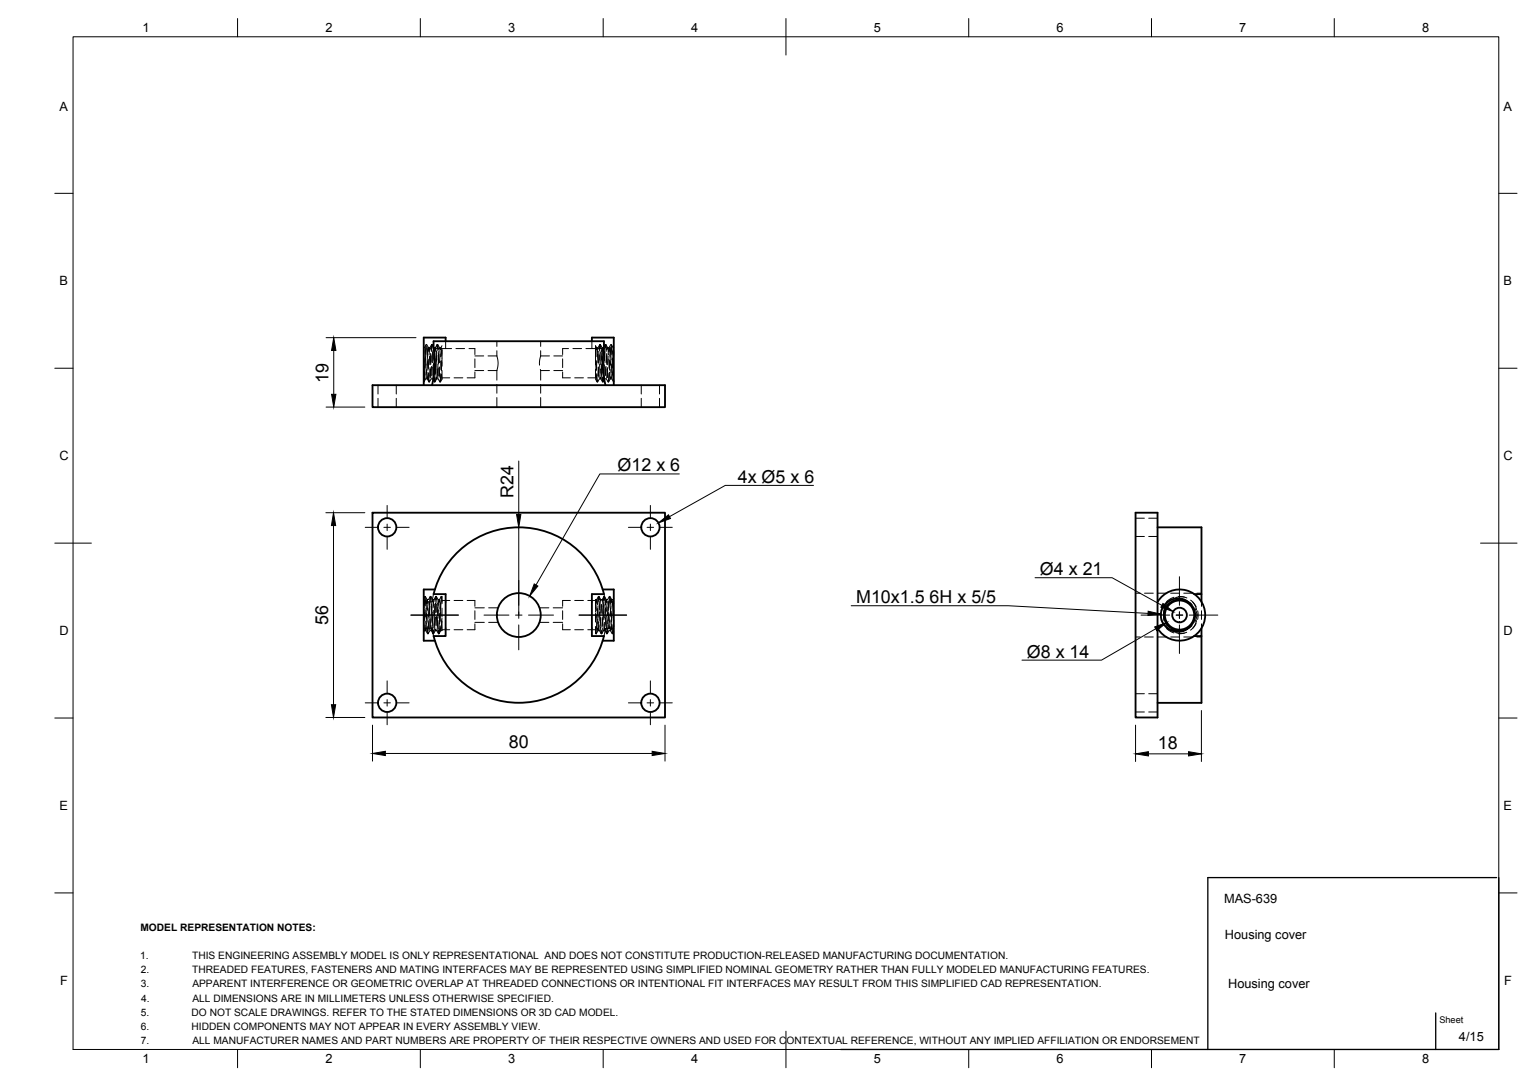
ISO-10303-21;
HEADER;
/* Generated by software containing ST-Developer
 * from STEP Tools, Inc. (www.steptools.com) 
 */

FILE_DESCRIPTION(
/* description */ ('Independent maintained push-to-latch/pull-to-reset mushroom-operator 
CAD. Two opposed spring-loaded ball detents in turned circular seats b
ias both travel stops; direct normally-closed bridge opens6mm when pre
ssed. Rounded palm/pull rim, captured head screw, removable detent clo
sures, native Coil spring families, insulated shared terminals and ord
inary machining features. Manual geometric states and ideal same-mater
ial spring-energy direction only; no electrical/safety certification, 
force/contact dynamics, wear, load or life rating. Requested blue/gray
 visual palette, not safety identification. External wiring/anchors an
d application engineering omitted.'),
/* implementation_level */ '2;1');

FILE_NAME(
/* name */ 'Housing cover.step',
/* time_stamp */ '2026-11-08T17:54:26-08:00',
/* author */ (''),
/* organization */ (''),
/* preprocessor_version */ 'ST-DEVELOPER v20.2',
/* originating_system */ 'Autodesk Translation Framework v15.17.0.0',
/* authorisation */ '');

FILE_SCHEMA (('AUTOMOTIVE_DESIGN { 1 0 10303 214 3 1 1 }'));
ENDSEC;

DATA;
#10=MECHANICAL_DESIGN_GEOMETRIC_PRESENTATION_REPRESENTATION('',(#191),#43980);
#157=SHAPE_REPRESENTATION_RELATIONSHIP('SRR','None',#44057,#174);
#174=ADVANCED_BREP_SHAPE_REPRESENTATION('',(#208),#43964);
#191=STYLED_ITEM('',(#44151),#208);
#208=MANIFOLD_SOLID_BREP('Body1',#11232);
#232=B_SPLINE_SURFACE_WITH_KNOTS('',3,3,((#23003,#23004,#23005,#23006,#23007,
#23008,#23009,#23010,#23011,#23012,#23013,#23014,#23015,#23016,#23017,#23018,
#23019,#23020,#23021,#23022,#23023,#23024,#23025,#23026,#23027,#23028,#23029,
#23030,#23031,#23032,#23033,#23034,#23035,#23036,#23037,#23038,#23039,#23040,
#23041,#23042,#23043,#23044,#23045,#23046,#23047,#23048,#23049,#23050,#23051),
(#23052,#23053,#23054,#23055,#23056,#23057,#23058,#23059,#23060,#23061,
#23062,#23063,#23064,#23065,#23066,#23067,#23068,#23069,#23070,#23071,#23072,
#23073,#23074,#23075,#23076,#23077,#23078,#23079,#23080,#23081,#23082,#23083,
#23084,#23085,#23086,#23087,#23088,#23089,#23090,#23091,#23092,#23093,#23094,
#23095,#23096,#23097,#23098,#23099,#23100),(#23101,#23102,#23103,#23104,
#23105,#23106,#23107,#23108,#23109,#23110,#23111,#23112,#23113,#23114,#23115,
#23116,#23117,#23118,#23119,#23120,#23121,#23122,#23123,#23124,#23125,#23126,
#23127,#23128,#23129,#23130,#23131,#23132,#23133,#23134,#23135,#23136,#23137,
#23138,#23139,#23140,#23141,#23142,#23143,#23144,#23145,#23146,#23147,#23148,
#23149),(#23150,#23151,#23152,#23153,#23154,#23155,#23156,#23157,#23158,
#23159,#23160,#23161,#23162,#23163,#23164,#23165,#23166,#23167,#23168,#23169,
#23170,#23171,#23172,#23173,#23174,#23175,#23176,#23177,#23178,#23179,#23180,
#23181,#23182,#23183,#23184,#23185,#23186,#23187,#23188,#23189,#23190,#23191,
#23192,#23193,#23194,#23195,#23196,#23197,#23198)),.UNSPECIFIED.,.F.,.F.,
 .F.,(4,4),(4,1,1,1,1,1,1,1,1,1,1,1,1,1,1,1,1,1,1,1,1,1,1,1,1,1,1,1,1,1,
1,1,1,1,1,1,1,1,1,1,1,1,1,1,1,1,4),(0.,0.0965329650085055),(11.852942864427,
12.3521979234545,12.851452982482,13.3507080415095,13.849963100537,14.3492181595645,
14.848473218592,15.3477282776195,15.846983336647,16.3462383956745,16.845493454702,
17.3447485137295,17.844003572757,18.3432586317845,18.842513690812,19.3417687498395,
19.841023808867,20.3402788678945,20.839533926922,21.3387889859495,21.838044044977,
22.3372991040045,22.836554163032,23.3358092220595,23.835064281087,24.3343193401145,
24.833574399142,25.3328294581695,25.832084517197,26.3313395762245,26.830594635252,
27.3298496942795,27.829104753307,28.3283598123345,28.827614871362,29.3268699303895,
29.826124989417,30.3253800484445,30.824635107472,31.3238901664995,31.823145225527,
32.3224002845545,32.821655343582,33.3209104026095,33.820165461637,34.3194205206645,
34.818675579692),.UNSPECIFIED.);
#233=B_SPLINE_SURFACE_WITH_KNOTS('',3,3,((#23385,#23386,#23387,#23388,#23389,
#23390,#23391,#23392,#23393,#23394,#23395,#23396,#23397,#23398,#23399,#23400,
#23401,#23402,#23403,#23404,#23405,#23406,#23407,#23408,#23409,#23410,#23411,
#23412,#23413,#23414,#23415,#23416,#23417,#23418,#23419,#23420,#23421,#23422,
#23423,#23424,#23425,#23426,#23427,#23428,#23429,#23430,#23431,#23432,#23433),
(#23434,#23435,#23436,#23437,#23438,#23439,#23440,#23441,#23442,#23443,
#23444,#23445,#23446,#23447,#23448,#23449,#23450,#23451,#23452,#23453,#23454,
#23455,#23456,#23457,#23458,#23459,#23460,#23461,#23462,#23463,#23464,#23465,
#23466,#23467,#23468,#23469,#23470,#23471,#23472,#23473,#23474,#23475,#23476,
#23477,#23478,#23479,#23480,#23481,#23482),(#23483,#23484,#23485,#23486,
#23487,#23488,#23489,#23490,#23491,#23492,#23493,#23494,#23495,#23496,#23497,
#23498,#23499,#23500,#23501,#23502,#23503,#23504,#23505,#23506,#23507,#23508,
#23509,#23510,#23511,#23512,#23513,#23514,#23515,#23516,#23517,#23518,#23519,
#23520,#23521,#23522,#23523,#23524,#23525,#23526,#23527,#23528,#23529,#23530,
#23531),(#23532,#23533,#23534,#23535,#23536,#23537,#23538,#23539,#23540,
#23541,#23542,#23543,#23544,#23545,#23546,#23547,#23548,#23549,#23550,#23551,
#23552,#23553,#23554,#23555,#23556,#23557,#23558,#23559,#23560,#23561,#23562,
#23563,#23564,#23565,#23566,#23567,#23568,#23569,#23570,#23571,#23572,#23573,
#23574,#23575,#23576,#23577,#23578,#23579,#23580)),.UNSPECIFIED.,.F.,.F.,
 .F.,(4,4),(4,1,1,1,1,1,1,1,1,1,1,1,1,1,1,1,1,1,1,1,1,1,1,1,1,1,1,1,1,1,
1,1,1,1,1,1,1,1,1,1,1,1,1,1,1,1,4),(0.,0.0965329650085055),(14.399609326548,
14.8988643855755,15.398119444603,15.8973745036305,16.396629562658,16.8958846216855,
17.395139680713,17.8943947397405,18.393649798768,18.8929048577955,19.392159916823,
19.8914149758505,20.390670034878,20.8899250939055,21.389180152933,21.8884352119605,
22.387690270988,22.8869453300155,23.386200389043,23.8854554480705,24.384710507098,
24.8839655661255,25.383220625153,25.8824756841805,26.381730743208,26.8809858022355,
27.380240861263,27.8794959202905,28.378750979318,28.8780060383455,29.377261097373,
29.8765161564005,30.375771215428,30.8750262744555,31.374281333483,31.8735363925105,
32.372791451538,32.8720465105655,33.371301569593,33.8705566286205,34.369811687648,
34.8690667466755,35.368321805703,35.8675768647305,36.366831923758,36.8660869827855,
37.365342041813),.UNSPECIFIED.);
#234=B_SPLINE_SURFACE_WITH_KNOTS('',3,3,((#23796,#23797,#23798,#23799,#23800,
#23801,#23802,#23803,#23804,#23805,#23806,#23807,#23808,#23809,#23810,#23811,
#23812,#23813,#23814,#23815,#23816,#23817,#23818,#23819,#23820,#23821,#23822,
#23823,#23824,#23825,#23826,#23827,#23828,#23829,#23830,#23831,#23832,#23833,
#23834,#23835,#23836,#23837,#23838,#23839,#23840,#23841,#23842,#23843,#23844),
(#23845,#23846,#23847,#23848,#23849,#23850,#23851,#23852,#23853,#23854,
#23855,#23856,#23857,#23858,#23859,#23860,#23861,#23862,#23863,#23864,#23865,
#23866,#23867,#23868,#23869,#23870,#23871,#23872,#23873,#23874,#23875,#23876,
#23877,#23878,#23879,#23880,#23881,#23882,#23883,#23884,#23885,#23886,#23887,
#23888,#23889,#23890,#23891,#23892,#23893),(#23894,#23895,#23896,#23897,
#23898,#23899,#23900,#23901,#23902,#23903,#23904,#23905,#23906,#23907,#23908,
#23909,#23910,#23911,#23912,#23913,#23914,#23915,#23916,#23917,#23918,#23919,
#23920,#23921,#23922,#23923,#23924,#23925,#23926,#23927,#23928,#23929,#23930,
#23931,#23932,#23933,#23934,#23935,#23936,#23937,#23938,#23939,#23940,#23941,
#23942),(#23943,#23944,#23945,#23946,#23947,#23948,#23949,#23950,#23951,
#23952,#23953,#23954,#23955,#23956,#23957,#23958,#23959,#23960,#23961,#23962,
#23963,#23964,#23965,#23966,#23967,#23968,#23969,#23970,#23971,#23972,#23973,
#23974,#23975,#23976,#23977,#23978,#23979,#23980,#23981,#23982,#23983,#23984,
#23985,#23986,#23987,#23988,#23989,#23990,#23991)),.UNSPECIFIED.,.F.,.F.,
 .F.,(4,4),(4,1,1,1,1,1,1,1,1,1,1,1,1,1,1,1,1,1,1,1,1,1,1,1,1,1,1,1,1,1,
1,1,1,1,1,1,1,1,1,1,1,1,1,1,1,1,4),(0.,0.0965329650085055),(11.852942864427,
12.3521979234545,12.851452982482,13.3507080415095,13.849963100537,14.3492181595645,
14.848473218592,15.3477282776195,15.846983336647,16.3462383956745,16.845493454702,
17.3447485137295,17.844003572757,18.3432586317845,18.842513690812,19.3417687498395,
19.841023808867,20.3402788678945,20.839533926922,21.3387889859495,21.838044044977,
22.3372991040045,22.836554163032,23.3358092220595,23.835064281087,24.3343193401145,
24.833574399142,25.3328294581695,25.832084517197,26.3313395762245,26.830594635252,
27.3298496942795,27.829104753307,28.3283598123345,28.827614871362,29.3268699303895,
29.826124989417,30.3253800484445,30.824635107472,31.3238901664995,31.823145225527,
32.3224002845545,32.821655343582,33.3209104026095,33.820165461637,34.3194205206645,
34.818675579692),.UNSPECIFIED.);
#235=B_SPLINE_SURFACE_WITH_KNOTS('',3,3,((#24178,#24179,#24180,#24181,#24182,
#24183,#24184,#24185,#24186,#24187,#24188,#24189,#24190,#24191,#24192,#24193,
#24194,#24195,#24196,#24197,#24198,#24199,#24200,#24201,#24202,#24203,#24204,
#24205,#24206,#24207,#24208,#24209,#24210,#24211,#24212,#24213,#24214,#24215,
#24216,#24217,#24218,#24219,#24220,#24221,#24222,#24223,#24224,#24225,#24226),
(#24227,#24228,#24229,#24230,#24231,#24232,#24233,#24234,#24235,#24236,
#24237,#24238,#24239,#24240,#24241,#24242,#24243,#24244,#24245,#24246,#24247,
#24248,#24249,#24250,#24251,#24252,#24253,#24254,#24255,#24256,#24257,#24258,
#24259,#24260,#24261,#24262,#24263,#24264,#24265,#24266,#24267,#24268,#24269,
#24270,#24271,#24272,#24273,#24274,#24275),(#24276,#24277,#24278,#24279,
#24280,#24281,#24282,#24283,#24284,#24285,#24286,#24287,#24288,#24289,#24290,
#24291,#24292,#24293,#24294,#24295,#24296,#24297,#24298,#24299,#24300,#24301,
#24302,#24303,#24304,#24305,#24306,#24307,#24308,#24309,#24310,#24311,#24312,
#24313,#24314,#24315,#24316,#24317,#24318,#24319,#24320,#24321,#24322,#24323,
#24324),(#24325,#24326,#24327,#24328,#24329,#24330,#24331,#24332,#24333,
#24334,#24335,#24336,#24337,#24338,#24339,#24340,#24341,#24342,#24343,#24344,
#24345,#24346,#24347,#24348,#24349,#24350,#24351,#24352,#24353,#24354,#24355,
#24356,#24357,#24358,#24359,#24360,#24361,#24362,#24363,#24364,#24365,#24366,
#24367,#24368,#24369,#24370,#24371,#24372,#24373)),.UNSPECIFIED.,.F.,.F.,
 .F.,(4,4),(4,1,1,1,1,1,1,1,1,1,1,1,1,1,1,1,1,1,1,1,1,1,1,1,1,1,1,1,1,1,
1,1,1,1,1,1,1,1,1,1,1,1,1,1,1,1,4),(0.,0.0965329650085055),(14.399609326548,
14.8988643855755,15.398119444603,15.8973745036305,16.396629562658,16.8958846216855,
17.395139680713,17.8943947397405,18.393649798768,18.8929048577955,19.392159916823,
19.8914149758505,20.390670034878,20.8899250939055,21.389180152933,21.8884352119605,
22.387690270988,22.8869453300155,23.386200389043,23.8854554480705,24.384710507098,
24.8839655661255,25.383220625153,25.8824756841805,26.381730743208,26.8809858022355,
27.380240861263,27.8794959202905,28.378750979318,28.8780060383455,29.377261097373,
29.8765161564005,30.375771215428,30.8750262744555,31.374281333483,31.8735363925105,
32.372791451538,32.8720465105655,33.371301569593,33.8705566286205,34.369811687648,
34.8690667466755,35.368321805703,35.8675768647305,36.366831923758,36.8660869827855,
37.365342041813),.UNSPECIFIED.);
#277=FACE_BOUND('',#1308,.T.);
#278=FACE_BOUND('',#1318,.T.);
#279=FACE_BOUND('',#1321,.T.);
#280=FACE_BOUND('',#1326,.T.);
#281=FACE_BOUND('',#1328,.T.);
#282=FACE_BOUND('',#1329,.T.);
#283=FACE_BOUND('',#1330,.T.);
#284=FACE_BOUND('',#1331,.T.);
#285=FACE_BOUND('',#1332,.T.);
#286=FACE_BOUND('',#1336,.T.);
#287=FACE_BOUND('',#1339,.T.);
#288=FACE_BOUND('',#1342,.T.);
#289=FACE_BOUND('',#1350,.T.);
#290=FACE_BOUND('',#1356,.T.);
#291=FACE_BOUND('',#1357,.T.);
#292=FACE_BOUND('',#1358,.T.);
#293=FACE_BOUND('',#1359,.T.);
#294=FACE_BOUND('',#1360,.T.);
#362=PLANE('',#11659);
#363=PLANE('',#11661);
#364=PLANE('',#11663);
#365=PLANE('',#11664);
#366=PLANE('',#11665);
#367=PLANE('',#11667);
#368=PLANE('',#11668);
#369=PLANE('',#11669);
#370=PLANE('',#11671);
#371=PLANE('',#11675);
#372=PLANE('',#11680);
#373=PLANE('',#11684);
#374=PLANE('',#11690);
#375=PLANE('',#11691);
#376=PLANE('',#11692);
#377=PLANE('',#11701);
#378=PLANE('',#11705);
#379=PLANE('',#11708);
#380=PLANE('',#11722);
#381=PLANE('',#11723);
#382=PLANE('',#11724);
#383=PLANE('',#11725);
#384=PLANE('',#11726);
#644=FACE_OUTER_BOUND('',#1285,.T.);
#645=FACE_OUTER_BOUND('',#1286,.T.);
#646=FACE_OUTER_BOUND('',#1287,.T.);
#647=FACE_OUTER_BOUND('',#1288,.T.);
#648=FACE_OUTER_BOUND('',#1289,.T.);
#649=FACE_OUTER_BOUND('',#1290,.T.);
#650=FACE_OUTER_BOUND('',#1291,.T.);
#651=FACE_OUTER_BOUND('',#1292,.T.);
#652=FACE_OUTER_BOUND('',#1293,.T.);
#653=FACE_OUTER_BOUND('',#1294,.T.);
#654=FACE_OUTER_BOUND('',#1295,.T.);
#655=FACE_OUTER_BOUND('',#1296,.T.);
#656=FACE_OUTER_BOUND('',#1297,.T.);
#657=FACE_OUTER_BOUND('',#1298,.T.);
#658=FACE_OUTER_BOUND('',#1299,.T.);
#659=FACE_OUTER_BOUND('',#1300,.T.);
#660=FACE_OUTER_BOUND('',#1301,.T.);
#661=FACE_OUTER_BOUND('',#1302,.T.);
#662=FACE_OUTER_BOUND('',#1303,.T.);
#663=FACE_OUTER_BOUND('',#1304,.T.);
#664=FACE_OUTER_BOUND('',#1305,.T.);
#665=FACE_OUTER_BOUND('',#1306,.T.);
#666=FACE_OUTER_BOUND('',#1307,.T.);
#667=FACE_OUTER_BOUND('',#1309,.T.);
#668=FACE_OUTER_BOUND('',#1310,.T.);
#669=FACE_OUTER_BOUND('',#1311,.T.);
#670=FACE_OUTER_BOUND('',#1312,.T.);
#671=FACE_OUTER_BOUND('',#1313,.T.);
#672=FACE_OUTER_BOUND('',#1314,.T.);
#673=FACE_OUTER_BOUND('',#1315,.T.);
#674=FACE_OUTER_BOUND('',#1316,.T.);
#675=FACE_OUTER_BOUND('',#1317,.T.);
#676=FACE_OUTER_BOUND('',#1319,.T.);
#677=FACE_OUTER_BOUND('',#1320,.T.);
#678=FACE_OUTER_BOUND('',#1322,.T.);
#679=FACE_OUTER_BOUND('',#1323,.T.);
#680=FACE_OUTER_BOUND('',#1324,.T.);
#681=FACE_OUTER_BOUND('',#1325,.T.);
#682=FACE_OUTER_BOUND('',#1327,.T.);
#683=FACE_OUTER_BOUND('',#1333,.T.);
#684=FACE_OUTER_BOUND('',#1334,.T.);
#685=FACE_OUTER_BOUND('',#1335,.T.);
#686=FACE_OUTER_BOUND('',#1337,.T.);
#687=FACE_OUTER_BOUND('',#1338,.T.);
#688=FACE_OUTER_BOUND('',#1340,.T.);
#689=FACE_OUTER_BOUND('',#1341,.T.);
#690=FACE_OUTER_BOUND('',#1343,.T.);
#691=FACE_OUTER_BOUND('',#1344,.T.);
#692=FACE_OUTER_BOUND('',#1345,.T.);
#693=FACE_OUTER_BOUND('',#1346,.T.);
#694=FACE_OUTER_BOUND('',#1347,.T.);
#695=FACE_OUTER_BOUND('',#1348,.T.);
#696=FACE_OUTER_BOUND('',#1349,.T.);
#697=FACE_OUTER_BOUND('',#1351,.T.);
#698=FACE_OUTER_BOUND('',#1352,.T.);
#699=FACE_OUTER_BOUND('',#1353,.T.);
#700=FACE_OUTER_BOUND('',#1354,.T.);
#701=FACE_OUTER_BOUND('',#1355,.T.);
#1285=EDGE_LOOP('',(#7755,#7756,#7757,#7758));
#1286=EDGE_LOOP('',(#7759,#7760,#7761,#7762));
#1287=EDGE_LOOP('',(#7763,#7764,#7765,#7766));
#1288=EDGE_LOOP('',(#7767,#7768,#7769,#7770));
#1289=EDGE_LOOP('',(#7771,#7772,#7773,#7774));
#1290=EDGE_LOOP('',(#7775,#7776,#7777,#7778));
#1291=EDGE_LOOP('',(#7779,#7780,#7781,#7782));
#1292=EDGE_LOOP('',(#7783,#7784,#7785,#7786));
#1293=EDGE_LOOP('',(#7787,#7788,#7789,#7790));
#1294=EDGE_LOOP('',(#7791,#7792,#7793,#7794));
#1295=EDGE_LOOP('',(#7795,#7796,#7797,#7798));
#1296=EDGE_LOOP('',(#7799,#7800,#7801,#7802));
#1297=EDGE_LOOP('',(#7803,#7804,#7805,#7806));
#1298=EDGE_LOOP('',(#7807,#7808,#7809,#7810));
#1299=EDGE_LOOP('',(#7811,#7812,#7813));
#1300=EDGE_LOOP('',(#7814,#7815,#7816));
#1301=EDGE_LOOP('',(#7817,#7818,#7819,#7820));
#1302=EDGE_LOOP('',(#7821,#7822,#7823,#7824));
#1303=EDGE_LOOP('',(#7825,#7826,#7827));
#1304=EDGE_LOOP('',(#7828,#7829,#7830,#7831));
#1305=EDGE_LOOP('',(#7832,#7833,#7834,#7835));
#1306=EDGE_LOOP('',(#7836,#7837,#7838));
#1307=EDGE_LOOP('',(#7839,#7840,#7841,#7842,#7843,#7844,#7845,#7846,#7847,
#7848,#7849,#7850));
#1308=EDGE_LOOP('',(#7851));
#1309=EDGE_LOOP('',(#7852,#7853));
#1310=EDGE_LOOP('',(#7854,#7855,#7856,#7857));
#1311=EDGE_LOOP('',(#7858,#7859,#7860,#7861,#7862,#7863,#7864,#7865,#7866,
#7867,#7868));
#1312=EDGE_LOOP('',(#7869,#7870,#7871,#7872,#7873,#7874,#7875,#7876,#7877,
#7878,#7879));
#1313=EDGE_LOOP('',(#7880,#7881,#7882,#7883));
#1314=EDGE_LOOP('',(#7884,#7885,#7886,#7887,#7888,#7889,#7890,#7891,#7892,
#7893,#7894));
#1315=EDGE_LOOP('',(#7895,#7896,#7897,#7898,#7899,#7900,#7901,#7902,#7903,
#7904,#7905));
#1316=EDGE_LOOP('',(#7906,#7907,#7908,#7909));
#1317=EDGE_LOOP('',(#7910,#7911,#7912,#7913));
#1318=EDGE_LOOP('',(#7914));
#1319=EDGE_LOOP('',(#7915,#7916,#7917,#7918));
#1320=EDGE_LOOP('',(#7919));
#1321=EDGE_LOOP('',(#7920));
#1322=EDGE_LOOP('',(#7921,#7922,#7923,#7924,#7925));
#1323=EDGE_LOOP('',(#7926,#7927,#7928,#7929,#7930,#7931,#7932,#7933,#7934,
#7935));
#1324=EDGE_LOOP('',(#7936,#7937));
#1325=EDGE_LOOP('',(#7938,#7939));
#1326=EDGE_LOOP('',(#7940,#7941,#7942,#7943));
#1327=EDGE_LOOP('',(#7944,#7945,#7946,#7947));
#1328=EDGE_LOOP('',(#7948));
#1329=EDGE_LOOP('',(#7949));
#1330=EDGE_LOOP('',(#7950));
#1331=EDGE_LOOP('',(#7951));
#1332=EDGE_LOOP('',(#7952,#7953,#7954,#7955,#7956,#7957,#7958,#7959));
#1333=EDGE_LOOP('',(#7960,#7961,#7962,#7963,#7964,#7965));
#1334=EDGE_LOOP('',(#7966,#7967,#7968,#7969));
#1335=EDGE_LOOP('',(#7970,#7971,#7972,#7973));
#1336=EDGE_LOOP('',(#7974));
#1337=EDGE_LOOP('',(#7975,#7976,#7977,#7978));
#1338=EDGE_LOOP('',(#7979));
#1339=EDGE_LOOP('',(#7980));
#1340=EDGE_LOOP('',(#7981,#7982,#7983,#7984,#7985,#7986,#7987));
#1341=EDGE_LOOP('',(#7988,#7989));
#1342=EDGE_LOOP('',(#7990,#7991,#7992,#7993));
#1343=EDGE_LOOP('',(#7994,#7995,#7996,#7997,#7998,#7999,#8000,#8001,#8002,
#8003));
#1344=EDGE_LOOP('',(#8004,#8005,#8006,#8007,#8008,#8009));
#1345=EDGE_LOOP('',(#8010,#8011,#8012,#8013));
#1346=EDGE_LOOP('',(#8014,#8015,#8016,#8017));
#1347=EDGE_LOOP('',(#8018,#8019,#8020,#8021));
#1348=EDGE_LOOP('',(#8022,#8023,#8024,#8025));
#1349=EDGE_LOOP('',(#8026,#8027,#8028,#8029,#8030,#8031,#8032,#8033,#8034,
#8035));
#1350=EDGE_LOOP('',(#8036,#8037));
#1351=EDGE_LOOP('',(#8038,#8039,#8040,#8041));
#1352=EDGE_LOOP('',(#8042,#8043,#8044,#8045));
#1353=EDGE_LOOP('',(#8046,#8047,#8048,#8049));
#1354=EDGE_LOOP('',(#8050,#8051,#8052,#8053));
#1355=EDGE_LOOP('',(#8054,#8055,#8056,#8057));
#1356=EDGE_LOOP('',(#8058));
#1357=EDGE_LOOP('',(#8059));
#1358=EDGE_LOOP('',(#8060));
#1359=EDGE_LOOP('',(#8061));
#1360=EDGE_LOOP('',(#8062));
#1847=CIRCLE('',#11638,0.4263);
#1848=CIRCLE('',#11641,0.4263);
#1849=CIRCLE('',#11643,0.4263);
#1850=CIRCLE('',#11646,0.4263);
#1851=CIRCLE('',#11648,0.5099);
#1852=CIRCLE('',#11652,0.5099);
#1853=CIRCLE('',#11654,0.5099);
#1854=CIRCLE('',#11658,0.5099);
#1855=CIRCLE('',#11660,0.7);
#1856=CIRCLE('',#11662,0.7);
#1857=CIRCLE('',#11666,0.7);
#1858=CIRCLE('',#11670,0.7);
#1859=CIRCLE('',#11672,2.4);
#1860=CIRCLE('',#11673,2.4);
#1861=CIRCLE('',#11674,0.6);
#1862=CIRCLE('',#11676,0.7);
#1863=CIRCLE('',#11681,0.4);
#1864=CIRCLE('',#11683,0.4);
#1865=CIRCLE('',#11685,0.2);
#1866=CIRCLE('',#11688,0.7);
#1867=CIRCLE('',#11689,0.7);
#1868=CIRCLE('',#11693,0.25);
#1869=CIRCLE('',#11694,0.25);
#1870=CIRCLE('',#11695,0.25);
#1871=CIRCLE('',#11696,0.25);
#1872=CIRCLE('',#11697,2.4);
#1873=CIRCLE('',#11698,2.4);
#1874=CIRCLE('',#11702,0.4);
#1875=CIRCLE('',#11704,0.4);
#1876=CIRCLE('',#11706,0.2);
#1877=CIRCLE('',#11709,0.7);
#1878=CIRCLE('',#11713,0.25);
#1879=CIRCLE('',#11715,0.25);
#1880=CIRCLE('',#11717,0.25);
#1881=CIRCLE('',#11719,0.25);
#1882=CIRCLE('',#11721,0.6);
#2228=B_SPLINE_CURVE_WITH_KNOTS('',3,(#22266,#22267,#22268,#22269,#22270,
#22271,#22272,#22273,#22274,#22275,#22276,#22277,#22278,#22279,#22280,#22281,
#22282,#22283,#22284),.UNSPECIFIED.,.F.,.F.,(4,3,3,3,3,3,4),(20.1579098629397,
20.4694574201275,20.968712479155,21.4679675381825,21.96722259721,22.4664776562375,
22.965732715265),.UNSPECIFIED.);
#2229=B_SPLINE_CURVE_WITH_KNOTS('',3,(#22287,#22288,#22289,#22290,#22291,
#22292,#22293,#22294,#22295,#22296,#22297,#22298,#22299,#22300,#22301,#22302,
#22303,#22304,#22305,#22306,#22307,#22308,#22309,#22310,#22311,#22312,#22313,
#22314,#22315,#22316,#22317),.UNSPECIFIED.,.F.,.F.,(4,3,3,3,3,3,3,3,3,3,
4),(-20.9439510239319,-20.4694574201275,-19.9702023611,-19.4709473020725,
-18.971692243045,-18.4724371840175,-17.97318212499,-17.4739270659625,-16.974672006935,
-16.4754169479075,-16.4213910178811),.UNSPECIFIED.);
#2230=B_SPLINE_CURVE_WITH_KNOTS('',3,(#22322,#22323,#22324,#22325,#22326,
#22327,#22328,#22329,#22330,#22331,#22332,#22333,#22334,#22335,#22336,#22337,
#22338,#22339,#22340,#22341,#22342,#22343,#22344,#22345,#22346,#22347,#22348,
#22349,#22350,#22351,#22352,#22353,#22354,#22355,#22356,#22357,#22358,#22359,
#22360,#22361,#22362,#22363,#22364),.UNSPECIFIED.,.F.,.F.,(4,3,3,3,3,3,
3,3,3,3,3,3,3,3,4),(13.8747245557602,13.97914165277,14.4783967117975,14.977651770825,
15.4769068298525,15.97616188888,16.4754169479075,16.974672006935,17.4739270659625,
17.97318212499,18.4724371840175,18.971692243045,19.4709473020725,19.9702023611,
20.1579098629397),.UNSPECIFIED.);
#2231=B_SPLINE_CURVE_WITH_KNOTS('',3,(#22365,#22366,#22367,#22368,#22369,
#22370,#22371,#22372,#22373,#22374,#22375,#22376,#22377,#22378,#22379,#22380,
#22381,#22382,#22383,#22384,#22385,#22386,#22387,#22388,#22389,#22390,#22391,
#22392,#22393,#22394,#22395,#22396,#22397,#22398,#22399,#22400,#22401,#22402,
#22403,#22404),.UNSPECIFIED.,.F.,.F.,(4,3,3,3,3,3,3,3,3,3,3,3,3,4),(-16.4213910178811,
-15.97616188888,-15.4769068298525,-14.977651770825,-14.4783967117975,-13.97914165277,
-13.4798865937425,-12.980631534715,-12.4813764756875,-11.98212141666,-11.4828663576325,
-10.983611298605,-10.4843562395775,-10.1382057107016),.UNSPECIFIED.);
#2232=B_SPLINE_CURVE_WITH_KNOTS('',3,(#22410,#22411,#22412,#22413,#22414,
#22415,#22416,#22417,#22418,#22419,#22420,#22421,#22422,#22423,#22424,#22425,
#22426,#22427,#22428,#22429,#22430,#22431,#22432,#22433,#22434),
 .UNSPECIFIED.,.F.,.F.,(4,3,3,3,3,3,3,3,4),(-3.85502040352197,-3.49478541319251,
-2.995530354165,-2.4962752951375,-1.99702023611001,-1.4977651770825,-0.998510118055002,
-0.499255059027501,0.),.UNSPECIFIED.);
#2233=B_SPLINE_CURVE_WITH_KNOTS('',3,(#22437,#22438,#22439,#22440,#22441,
#22442,#22443,#22444,#22445,#22446,#22447,#22448,#22449,#22450,#22451,#22452,
#22453,#22454,#22455,#22456,#22457,#22458,#22459,#22460,#22461,#22462,#22463,
#22464,#22465,#22466,#22467,#22468,#22469,#22470,#22471,#22472,#22473),
 .UNSPECIFIED.,.F.,.F.,(4,3,3,3,3,3,3,3,3,3,3,3,4),(2.02178169133306,2.4962752951375,
2.99553035416501,3.49478541319251,3.99404047222001,4.49329553124751,4.99255059027501,
5.49180564930251,5.99106070833001,6.49031576735751,6.98957082638501,7.48882588541252,
7.59153924858057),.UNSPECIFIED.);
#2234=B_SPLINE_CURVE_WITH_KNOTS('',3,(#22479,#22480,#22481,#22482,#22483,
#22484,#22485,#22486,#22487,#22488,#22489,#22490,#22491,#22492,#22493,#22494,
#22495,#22496,#22497),.UNSPECIFIED.,.F.,.F.,(4,3,3,3,3,3,4),(20.1579098629397,
20.4694574201275,20.968712479155,21.4679675381825,21.96722259721,22.4664776562375,
22.965732715265),.UNSPECIFIED.);
#2235=B_SPLINE_CURVE_WITH_KNOTS('',3,(#22500,#22501,#22502,#22503,#22504,
#22505,#22506,#22507,#22508,#22509,#22510,#22511,#22512,#22513,#22514,#22515,
#22516,#22517,#22518,#22519,#22520,#22521,#22522,#22523,#22524,#22525,#22526,
#22527,#22528,#22529,#22530),.UNSPECIFIED.,.F.,.F.,(4,3,3,3,3,3,3,3,3,3,
4),(-20.9439510239319,-20.4694574201275,-19.9702023611,-19.4709473020725,
-18.971692243045,-18.4724371840175,-17.97318212499,-17.4739270659625,-16.974672006935,
-16.4754169479075,-16.4213910178811),.UNSPECIFIED.);
#2236=B_SPLINE_CURVE_WITH_KNOTS('',3,(#22535,#22536,#22537,#22538,#22539,
#22540,#22541,#22542,#22543,#22544,#22545,#22546,#22547,#22548,#22549,#22550,
#22551,#22552,#22553,#22554,#22555,#22556,#22557,#22558,#22559,#22560,#22561,
#22562,#22563,#22564,#22565,#22566,#22567,#22568,#22569,#22570,#22571,#22572,
#22573,#22574,#22575,#22576,#22577),.UNSPECIFIED.,.F.,.F.,(4,3,3,3,3,3,
3,3,3,3,3,3,3,3,4),(13.8747245557602,13.97914165277,14.4783967117975,14.977651770825,
15.4769068298525,15.97616188888,16.4754169479075,16.974672006935,17.4739270659625,
17.97318212499,18.4724371840175,18.971692243045,19.4709473020725,19.9702023611,
20.1579098629397),.UNSPECIFIED.);
#2237=B_SPLINE_CURVE_WITH_KNOTS('',3,(#22578,#22579,#22580,#22581,#22582,
#22583,#22584,#22585,#22586,#22587,#22588,#22589,#22590,#22591,#22592,#22593,
#22594,#22595,#22596,#22597,#22598,#22599,#22600,#22601,#22602,#22603,#22604,
#22605,#22606,#22607,#22608,#22609,#22610,#22611,#22612,#22613,#22614,#22615,
#22616,#22617),.UNSPECIFIED.,.F.,.F.,(4,3,3,3,3,3,3,3,3,3,3,3,3,4),(-16.4213910178811,
-15.97616188888,-15.4769068298525,-14.977651770825,-14.4783967117975,-13.97914165277,
-13.4798865937425,-12.980631534715,-12.4813764756875,-11.98212141666,-11.4828663576325,
-10.983611298605,-10.4843562395775,-10.1382057107016),.UNSPECIFIED.);
#2238=B_SPLINE_CURVE_WITH_KNOTS('',3,(#22623,#22624,#22625,#22626,#22627,
#22628,#22629,#22630,#22631,#22632,#22633,#22634,#22635,#22636,#22637,#22638,
#22639,#22640,#22641,#22642,#22643,#22644,#22645,#22646,#22647),
 .UNSPECIFIED.,.F.,.F.,(4,3,3,3,3,3,3,3,4),(-3.85502040352197,-3.49478541319251,
-2.995530354165,-2.4962752951375,-1.99702023611001,-1.4977651770825,-0.998510118055002,
-0.499255059027501,0.),.UNSPECIFIED.);
#2239=B_SPLINE_CURVE_WITH_KNOTS('',3,(#22650,#22651,#22652,#22653,#22654,
#22655,#22656,#22657,#22658,#22659,#22660,#22661,#22662,#22663,#22664,#22665,
#22666,#22667,#22668,#22669,#22670,#22671,#22672,#22673,#22674,#22675,#22676,
#22677,#22678,#22679,#22680,#22681,#22682,#22683,#22684,#22685,#22686),
 .UNSPECIFIED.,.F.,.F.,(4,3,3,3,3,3,3,3,3,3,3,3,4),(2.02178169133306,2.4962752951375,
2.99553035416501,3.49478541319251,3.99404047222001,4.49329553124751,4.99255059027501,
5.49180564930251,5.99106070833001,6.49031576735751,6.98957082638501,7.48882588541252,
7.59153924858057),.UNSPECIFIED.);
#2240=B_SPLINE_CURVE_WITH_KNOTS('',3,(#22692,#22693,#22694,#22695),
 .UNSPECIFIED.,.F.,.F.,(4,4),(34.5575191894877,34.818675579692),
 .UNSPECIFIED.);
#2241=B_SPLINE_CURVE_WITH_KNOTS('',3,(#22698,#22699,#22700,#22701,#22702),
 .UNSPECIFIED.,.F.,.F.,(4,1,4),(34.5575191894877,34.8690667466755,35.3435603504799),
 .UNSPECIFIED.);
#2242=B_SPLINE_CURVE_WITH_KNOTS('',3,(#22707,#22708,#22709,#22710,#22711,
#22712,#22713,#22714,#22715,#22716,#22717,#22718,#22719,#22720,#22721,#22722,
#22723),.UNSPECIFIED.,.F.,.F.,(4,1,1,1,1,1,1,1,1,1,1,1,1,1,4),(28.2743338823081,
28.3283598123345,28.827614871362,29.3268699303895,29.826124989417,30.3253800484445,
30.824635107472,31.3238901664995,31.823145225527,32.3224002845545,32.821655343582,
33.3209104026095,33.820165461637,34.3194205206645,34.5575191894877),
 .UNSPECIFIED.);
#2243=B_SPLINE_CURVE_WITH_KNOTS('',3,(#22724,#22725,#22726,#22727,#22728,
#22729,#22730,#22731,#22732,#22733,#22734,#22735,#22736,#22737,#22738,#22739,
#22740),.UNSPECIFIED.,.F.,.F.,(4,1,1,1,1,1,1,1,1,1,1,1,1,1,4),(28.2743338823081,
28.378750979318,28.8780060383455,29.377261097373,29.8765161564005,30.375771215428,
30.8750262744555,31.374281333483,31.8735363925105,32.372791451538,32.8720465105655,
33.371301569593,33.8705566286205,34.369811687648,34.5575191894877),
 .UNSPECIFIED.);
#2244=B_SPLINE_CURVE_WITH_KNOTS('',3,(#22745,#22746,#22747,#22748,#22749,
#22750,#22751,#22752,#22753,#22754,#22755,#22756,#22757,#22758,#22759,#22760),
 .UNSPECIFIED.,.F.,.F.,(4,1,1,1,1,1,1,1,1,1,1,1,1,4),(21.9911485751285,
22.3372991040045,22.836554163032,23.3358092220595,23.835064281087,24.3343193401145,
24.833574399142,25.3328294581695,25.832084517197,26.3313395762245,26.830594635252,
27.3298496942795,27.829104753307,28.2743338823081),.UNSPECIFIED.);
#2245=B_SPLINE_CURVE_WITH_KNOTS('',3,(#22761,#22762,#22763,#22764,#22765,
#22766,#22767,#22768,#22769,#22770,#22771,#22772,#22773,#22774,#22775,#22776),
 .UNSPECIFIED.,.F.,.F.,(4,1,1,1,1,1,1,1,1,1,1,1,1,4),(21.9911485751285,
22.387690270988,22.8869453300155,23.386200389043,23.8854554480705,24.384710507098,
24.8839655661255,25.383220625153,25.8824756841805,26.381730743208,26.8809858022355,
27.380240861263,27.8794959202905,28.2743338823081),.UNSPECIFIED.);
#2246=B_SPLINE_CURVE_WITH_KNOTS('',3,(#22782,#22783,#22784,#22785,#22786,
#22787),.UNSPECIFIED.,.F.,.F.,(4,1,1,4),(14.399609326548,14.8988643855755,
15.398119444603,15.707963267949),.UNSPECIFIED.);
#2247=B_SPLINE_CURVE_WITH_KNOTS('',3,(#22790,#22791,#22792,#22793,#22794,
#22795,#22796),.UNSPECIFIED.,.F.,.F.,(4,1,1,1,4),(13.8747245557601,14.3492181595645,
14.848473218592,15.3477282776195,15.707963267949),.UNSPECIFIED.);
#2248=B_SPLINE_CURVE_WITH_KNOTS('',3,(#22802,#22803,#22804,#22805),
 .UNSPECIFIED.,.F.,.F.,(4,4),(34.5575191894877,34.818675579692),
 .UNSPECIFIED.);
#2249=B_SPLINE_CURVE_WITH_KNOTS('',3,(#22808,#22809,#22810,#22811,#22812),
 .UNSPECIFIED.,.F.,.F.,(4,1,4),(34.5575191894877,34.8690667466755,35.3435603504799),
 .UNSPECIFIED.);
#2250=B_SPLINE_CURVE_WITH_KNOTS('',3,(#22817,#22818,#22819,#22820,#22821,
#22822,#22823,#22824,#22825,#22826,#22827,#22828,#22829,#22830,#22831,#22832,
#22833),.UNSPECIFIED.,.F.,.F.,(4,1,1,1,1,1,1,1,1,1,1,1,1,1,4),(28.2743338823081,
28.3283598123345,28.827614871362,29.3268699303895,29.826124989417,30.3253800484445,
30.824635107472,31.3238901664995,31.823145225527,32.3224002845545,32.821655343582,
33.3209104026095,33.820165461637,34.3194205206645,34.5575191894877),
 .UNSPECIFIED.);
#2251=B_SPLINE_CURVE_WITH_KNOTS('',3,(#22834,#22835,#22836,#22837,#22838,
#22839,#22840,#22841,#22842,#22843,#22844,#22845,#22846,#22847,#22848,#22849,
#22850),.UNSPECIFIED.,.F.,.F.,(4,1,1,1,1,1,1,1,1,1,1,1,1,1,4),(28.2743338823081,
28.378750979318,28.8780060383455,29.377261097373,29.8765161564005,30.375771215428,
30.8750262744555,31.374281333483,31.8735363925105,32.372791451538,32.8720465105655,
33.371301569593,33.8705566286205,34.369811687648,34.5575191894877),
 .UNSPECIFIED.);
#2252=B_SPLINE_CURVE_WITH_KNOTS('',3,(#22855,#22856,#22857,#22858,#22859,
#22860,#22861,#22862,#22863,#22864,#22865,#22866,#22867,#22868,#22869,#22870),
 .UNSPECIFIED.,.F.,.F.,(4,1,1,1,1,1,1,1,1,1,1,1,1,4),(21.9911485751285,
22.3372991040045,22.836554163032,23.3358092220595,23.835064281087,24.3343193401145,
24.833574399142,25.3328294581695,25.832084517197,26.3313395762245,26.830594635252,
27.3298496942795,27.829104753307,28.2743338823081),.UNSPECIFIED.);
#2253=B_SPLINE_CURVE_WITH_KNOTS('',3,(#22871,#22872,#22873,#22874,#22875,
#22876,#22877,#22878,#22879,#22880,#22881,#22882,#22883,#22884,#22885,#22886),
 .UNSPECIFIED.,.F.,.F.,(4,1,1,1,1,1,1,1,1,1,1,1,1,4),(21.9911485751285,
22.387690270988,22.8869453300155,23.386200389043,23.8854554480705,24.384710507098,
24.8839655661255,25.383220625153,25.8824756841805,26.381730743208,26.8809858022355,
27.380240861263,27.8794959202905,28.2743338823081),.UNSPECIFIED.);
#2254=B_SPLINE_CURVE_WITH_KNOTS('',3,(#22892,#22893,#22894,#22895,#22896,
#22897),.UNSPECIFIED.,.F.,.F.,(4,1,1,4),(14.399609326548,14.8988643855755,
15.398119444603,15.707963267949),.UNSPECIFIED.);
#2255=B_SPLINE_CURVE_WITH_KNOTS('',3,(#22900,#22901,#22902,#22903,#22904,
#22905,#22906),.UNSPECIFIED.,.F.,.F.,(4,1,1,1,4),(13.8747245557601,14.3492181595645,
14.848473218592,15.3477282776195,15.707963267949),.UNSPECIFIED.);
#2256=B_SPLINE_CURVE_WITH_KNOTS('',3,(#22969,#22970,#22971,#22972,#22973,
#22974,#22975,#22976,#22977,#22978,#22979,#22980,#22981,#22982,#22983,#22984,
#22985),.UNSPECIFIED.,.F.,.F.,(4,1,1,1,1,1,1,1,1,1,1,1,1,1,4),(15.707963267949,
15.846983336647,16.3462383956745,16.845493454702,17.3447485137295,17.844003572757,
18.3432586317845,18.842513690812,19.3417687498395,19.841023808867,20.3402788678945,
20.839533926922,21.3387889859495,21.838044044977,21.9911485751285),
 .UNSPECIFIED.);
#2257=B_SPLINE_CURVE_WITH_KNOTS('',3,(#22986,#22987,#22988,#22989,#22990,
#22991,#22992,#22993,#22994,#22995,#22996,#22997,#22998,#22999,#23000,#23001,
#23002),.UNSPECIFIED.,.F.,.F.,(4,1,1,1,1,1,1,1,1,1,1,1,1,1,4),(15.707963267949,
15.8973745036305,16.396629562658,16.8958846216855,17.395139680713,17.8943947397405,
18.393649798768,18.8929048577955,19.392159916823,19.8914149758505,20.390670034878,
20.8899250939055,21.389180152933,21.8884352119605,21.9911485751285),
 .UNSPECIFIED.);
#2258=B_SPLINE_CURVE_WITH_KNOTS('',3,(#23199,#23200,#23201,#23202,#23203,
#23204,#23205,#23206,#23207,#23208,#23209,#23210,#23211,#23212,#23213,#23214,
#23215,#23216,#23217,#23218,#23219,#23220,#23221,#23222,#23223,#23224,#23225,
#23226,#23227,#23228,#23229,#23230,#23231,#23232,#23233,#23234,#23235,#23236,
#23237,#23238,#23239,#23240,#23241,#23242,#23243,#23244,#23245,#23246,#23247,
#23248,#23249,#23250,#23251,#23252,#23253,#23254,#23255,#23256,#23257,#23258,
#23259,#23260,#23261,#23262,#23263,#23264,#23265,#23266,#23267,#23268,#23269,
#23270,#23271),.UNSPECIFIED.,.F.,.F.,(4,3,3,3,3,3,3,3,3,3,3,3,3,3,3,3,3,
3,3,3,3,3,3,3,4),(-0.950777871811465,-0.888334407370769,-0.851051814776991,
-0.82737904373313,-0.764191528890905,-0.727096293545134,-0.707864357405063,
-0.701004014048681,-0.624532510230306,-0.548715306176616,-0.528886751702636,
-0.51335217329456,-0.460845815077925,-0.386468184274459,-0.349072714542667,
-0.331943455188318,-0.259671363135132,-0.230659644409349,-0.19743434794885,
-0.175120034180883,-0.157580682039417,-0.0841021758717334,-0.0150413926252008,
-0.0106236697040495,0.),.UNSPECIFIED.);
#2259=B_SPLINE_CURVE_WITH_KNOTS('',3,(#23272,#23273,#23274,#23275,#23276,
#23277,#23278,#23279,#23280,#23281,#23282,#23283,#23284,#23285,#23286,#23287,
#23288,#23289,#23290,#23291,#23292,#23293,#23294,#23295,#23296,#23297,#23298,
#23299,#23300,#23301,#23302,#23303,#23304,#23305,#23306,#23307,#23308,#23309,
#23310,#23311,#23312,#23313,#23314,#23315,#23316,#23317,#23318,#23319,#23320,
#23321,#23322,#23323,#23324,#23325,#23326,#23327,#23328,#23329,#23330,#23331,
#23332,#23333,#23334,#23335,#23336,#23337,#23338,#23339,#23340,#23341),
 .UNSPECIFIED.,.F.,.F.,(4,3,3,3,3,3,3,3,3,3,3,3,3,3,3,3,3,3,3,3,3,3,3,4),
(0.,0.0695167991119783,0.140212658431775,0.162172470483188,0.179979408684031,
0.219498223261391,0.291822018016311,0.337745303611425,0.355228583776568,
0.429645631566202,0.449180111380345,0.509263572656178,0.525649154341391,
0.601088264154331,0.677503858556246,0.688874999321038,0.709603483853625,
0.730479306054779,0.782399641108501,0.820902701806524,0.845385896033558,
0.924612288143001,0.938160646269666,0.950777871811463),.UNSPECIFIED.);
#2260=B_SPLINE_CURVE_WITH_KNOTS('',3,(#23342,#23343,#23344,#23345,#23346,
#23347,#23348,#23349,#23350,#23351,#23352,#23353,#23354,#23355,#23356,#23357,
#23358,#23359,#23360,#23361,#23362,#23363,#23364,#23365,#23366,#23367,#23368,
#23369,#23370,#23371,#23372,#23373,#23374,#23375,#23376,#23377,#23378,#23379,
#23380,#23381,#23382,#23383,#23384),.UNSPECIFIED.,.F.,.F.,(4,3,3,3,3,3,
3,3,3,3,3,3,3,3,4),(-10.1382057107016,-9.98510118055001,-9.48584612152251,
-8.98659106249501,-8.48733600346751,-7.98808094444001,-7.48882588541251,
-6.98957082638501,-6.49031576735751,-5.99106070833001,-5.49180564930251,
-4.99255059027501,-4.49329553124751,-3.99404047222001,-3.85502040352197),
 .UNSPECIFIED.);
#2261=B_SPLINE_CURVE_WITH_KNOTS('',3,(#23581,#23582,#23583,#23584,#23585,
#23586,#23587,#23588,#23589,#23590,#23591,#23592,#23593,#23594,#23595,#23596,
#23597,#23598,#23599,#23600,#23601,#23602,#23603,#23604,#23605,#23606,#23607,
#23608,#23609,#23610,#23611,#23612,#23613,#23614,#23615,#23616,#23617,#23618,
#23619,#23620,#23621,#23622,#23623,#23624,#23625,#23626,#23627,#23628,#23629,
#23630,#23631,#23632,#23633,#23634,#23635,#23636,#23637,#23638,#23639,#23640,
#23641,#23642,#23643,#23644,#23645,#23646,#23647,#23648,#23649,#23650),
 .UNSPECIFIED.,.F.,.F.,(4,3,3,3,3,3,3,3,3,3,3,3,3,3,3,3,3,3,3,3,3,3,3,4),
(-0.954382097139049,-0.899410408801335,-0.859358635307587,-0.836685957905282,
-0.785590650846737,-0.75140161257743,-0.734495343788191,-0.662158982507963,
-0.588787990221564,-0.570217280263643,-0.551422718402641,-0.504011712732237,
-0.443843717567291,-0.393584703400901,-0.372143080358795,-0.295059059270718,
-0.263339732072452,-0.224912725821683,-0.201648013648112,-0.183362315801792,
-0.105092336646239,-0.0261711118220366,-0.0126626251736613,0.),
 .UNSPECIFIED.);
#2262=B_SPLINE_CURVE_WITH_KNOTS('',3,(#23651,#23652,#23653,#23654,#23655,
#23656,#23657,#23658,#23659,#23660,#23661,#23662,#23663,#23664,#23665,#23666,
#23667,#23668,#23669,#23670,#23671,#23672,#23673,#23674,#23675,#23676,#23677,
#23678,#23679,#23680,#23681,#23682,#23683,#23684,#23685,#23686,#23687,#23688,
#23689,#23690),.UNSPECIFIED.,.F.,.F.,(4,3,3,3,3,3,3,3,3,3,3,3,3,4),(7.59153924858057,
7.98808094444002,8.48733600346752,8.98659106249502,9.48584612152252,9.98510118055002,
10.4843562395775,10.983611298605,11.4828663576325,11.98212141666,12.4813764756875,
12.980631534715,13.4798865937425,13.8747245557602),.UNSPECIFIED.);
#2263=B_SPLINE_CURVE_WITH_KNOTS('',3,(#23691,#23692,#23693,#23694,#23695,
#23696,#23697,#23698,#23699,#23700,#23701,#23702,#23703,#23704,#23705,#23706,
#23707,#23708,#23709,#23710,#23711,#23712,#23713,#23714,#23715,#23716,#23717,
#23718,#23719,#23720,#23721,#23722,#23723,#23724,#23725,#23726,#23727,#23728,
#23729,#23730,#23731,#23732,#23733,#23734,#23735,#23736,#23737,#23738,#23739,
#23740,#23741,#23742,#23743,#23744,#23745,#23746,#23747,#23748,#23749,#23750,
#23751,#23752,#23753,#23754,#23755,#23756,#23757,#23758,#23759,#23760),
 .UNSPECIFIED.,.F.,.F.,(4,3,3,3,3,3,3,3,3,3,3,3,3,3,3,3,3,3,3,3,3,3,3,4),
(0.,0.079016546580938,0.157641122394585,0.183993443720854,0.207891281656444,
0.251131687956984,0.328243571587973,0.374168384090539,0.397099877179475,
0.472026294619315,0.492301725366521,0.550056206928688,0.568103933485432,
0.584735378149958,0.65759847554391,0.72331965161519,0.743939980328521,0.763679188248337,
0.809798919188833,0.846311488438111,0.867561854219163,0.937273050771799,
0.943726018375008,0.954382097139032),.UNSPECIFIED.);
#2264=B_SPLINE_CURVE_WITH_KNOTS('',3,(#23762,#23763,#23764,#23765,#23766,
#23767,#23768,#23769,#23770,#23771,#23772,#23773,#23774,#23775,#23776,#23777,
#23778),.UNSPECIFIED.,.F.,.F.,(4,1,1,1,1,1,1,1,1,1,1,1,1,1,4),(15.707963267949,
15.846983336647,16.3462383956745,16.845493454702,17.3447485137295,17.844003572757,
18.3432586317845,18.842513690812,19.3417687498395,19.841023808867,20.3402788678945,
20.839533926922,21.3387889859495,21.838044044977,21.9911485751285),
 .UNSPECIFIED.);
#2265=B_SPLINE_CURVE_WITH_KNOTS('',3,(#23779,#23780,#23781,#23782,#23783,
#23784,#23785,#23786,#23787,#23788,#23789,#23790,#23791,#23792,#23793,#23794,
#23795),.UNSPECIFIED.,.F.,.F.,(4,1,1,1,1,1,1,1,1,1,1,1,1,1,4),(15.707963267949,
15.8973745036305,16.396629562658,16.8958846216855,17.395139680713,17.8943947397405,
18.393649798768,18.8929048577955,19.392159916823,19.8914149758505,20.390670034878,
20.8899250939055,21.389180152933,21.8884352119605,21.9911485751285),
 .UNSPECIFIED.);
#2266=B_SPLINE_CURVE_WITH_KNOTS('',3,(#23992,#23993,#23994,#23995,#23996,
#23997,#23998,#23999,#24000,#24001,#24002,#24003,#24004,#24005,#24006,#24007,
#24008,#24009,#24010,#24011,#24012,#24013,#24014,#24015,#24016,#24017,#24018,
#24019,#24020,#24021,#24022,#24023,#24024,#24025,#24026,#24027,#24028,#24029,
#24030,#24031,#24032,#24033,#24034,#24035,#24036,#24037,#24038,#24039,#24040,
#24041,#24042,#24043,#24044,#24045,#24046,#24047,#24048,#24049,#24050,#24051,
#24052,#24053,#24054,#24055,#24056,#24057,#24058,#24059,#24060,#24061,#24062,
#24063,#24064),.UNSPECIFIED.,.F.,.F.,(4,3,3,3,3,3,3,3,3,3,3,3,3,3,3,3,3,
3,3,3,3,3,3,3,4),(-0.950777871811465,-0.888334407370769,-0.851051814776991,
-0.82737904373313,-0.764191528890905,-0.727096293545134,-0.707864357405063,
-0.701004014048681,-0.624532510230306,-0.548715306176616,-0.528886751702636,
-0.51335217329456,-0.460845815077925,-0.386468184274459,-0.349072714542667,
-0.331943455188318,-0.259671363135132,-0.230659644409349,-0.19743434794885,
-0.175120034180883,-0.157580682039417,-0.0841021758717334,-0.0150413926252008,
-0.0106236697040495,0.),.UNSPECIFIED.);
#2267=B_SPLINE_CURVE_WITH_KNOTS('',3,(#24065,#24066,#24067,#24068,#24069,
#24070,#24071,#24072,#24073,#24074,#24075,#24076,#24077,#24078,#24079,#24080,
#24081,#24082,#24083,#24084,#24085,#24086,#24087,#24088,#24089,#24090,#24091,
#24092,#24093,#24094,#24095,#24096,#24097,#24098,#24099,#24100,#24101,#24102,
#24103,#24104,#24105,#24106,#24107,#24108,#24109,#24110,#24111,#24112,#24113,
#24114,#24115,#24116,#24117,#24118,#24119,#24120,#24121,#24122,#24123,#24124,
#24125,#24126,#24127,#24128,#24129,#24130,#24131,#24132,#24133,#24134),
 .UNSPECIFIED.,.F.,.F.,(4,3,3,3,3,3,3,3,3,3,3,3,3,3,3,3,3,3,3,3,3,3,3,4),
(0.,0.0695167991119783,0.140212658431775,0.162172470483188,0.179979408684031,
0.219498223261391,0.291822018016311,0.337745303611425,0.355228583776568,
0.429645631566202,0.449180111380345,0.509263572656178,0.525649154341391,
0.601088264154331,0.677503858556246,0.688874999321038,0.709603483853625,
0.730479306054779,0.782399641108501,0.820902701806524,0.845385896033558,
0.924612288143001,0.938160646269666,0.950777871811463),.UNSPECIFIED.);
#2268=B_SPLINE_CURVE_WITH_KNOTS('',3,(#24135,#24136,#24137,#24138,#24139,
#24140,#24141,#24142,#24143,#24144,#24145,#24146,#24147,#24148,#24149,#24150,
#24151,#24152,#24153,#24154,#24155,#24156,#24157,#24158,#24159,#24160,#24161,
#24162,#24163,#24164,#24165,#24166,#24167,#24168,#24169,#24170,#24171,#24172,
#24173,#24174,#24175,#24176,#24177),.UNSPECIFIED.,.F.,.F.,(4,3,3,3,3,3,
3,3,3,3,3,3,3,3,4),(-10.1382057107016,-9.98510118055001,-9.48584612152251,
-8.98659106249501,-8.48733600346751,-7.98808094444001,-7.48882588541251,
-6.98957082638501,-6.49031576735751,-5.99106070833001,-5.49180564930251,
-4.99255059027501,-4.49329553124751,-3.99404047222001,-3.85502040352197),
 .UNSPECIFIED.);
#2269=B_SPLINE_CURVE_WITH_KNOTS('',3,(#24374,#24375,#24376,#24377,#24378,
#24379,#24380,#24381,#24382,#24383,#24384,#24385,#24386,#24387,#24388,#24389,
#24390,#24391,#24392,#24393,#24394,#24395,#24396,#24397,#24398,#24399,#24400,
#24401,#24402,#24403,#24404,#24405,#24406,#24407,#24408,#24409,#24410,#24411,
#24412,#24413,#24414,#24415,#24416,#24417,#24418,#24419,#24420,#24421,#24422,
#24423,#24424,#24425,#24426,#24427,#24428,#24429,#24430,#24431,#24432,#24433,
#24434,#24435,#24436,#24437,#24438,#24439,#24440,#24441,#24442,#24443),
 .UNSPECIFIED.,.F.,.F.,(4,3,3,3,3,3,3,3,3,3,3,3,3,3,3,3,3,3,3,3,3,3,3,4),
(-0.954382097139049,-0.899410408801335,-0.859358635307587,-0.836685957905282,
-0.785590650846737,-0.75140161257743,-0.734495343788191,-0.662158982507963,
-0.588787990221564,-0.570217280263643,-0.551422718402641,-0.504011712732237,
-0.443843717567291,-0.393584703400901,-0.372143080358795,-0.295059059270718,
-0.263339732072452,-0.224912725821683,-0.201648013648112,-0.183362315801792,
-0.105092336646239,-0.0261711118220366,-0.0126626251736613,0.),
 .UNSPECIFIED.);
#2270=B_SPLINE_CURVE_WITH_KNOTS('',3,(#24444,#24445,#24446,#24447,#24448,
#24449,#24450,#24451,#24452,#24453,#24454,#24455,#24456,#24457,#24458,#24459,
#24460,#24461,#24462,#24463,#24464,#24465,#24466,#24467,#24468,#24469,#24470,
#24471,#24472,#24473,#24474,#24475,#24476,#24477,#24478,#24479,#24480,#24481,
#24482,#24483),.UNSPECIFIED.,.F.,.F.,(4,3,3,3,3,3,3,3,3,3,3,3,3,4),(7.59153924858057,
7.98808094444002,8.48733600346752,8.98659106249502,9.48584612152252,9.98510118055002,
10.4843562395775,10.983611298605,11.4828663576325,11.98212141666,12.4813764756875,
12.980631534715,13.4798865937425,13.8747245557602),.UNSPECIFIED.);
#2271=B_SPLINE_CURVE_WITH_KNOTS('',3,(#24484,#24485,#24486,#24487,#24488,
#24489,#24490,#24491,#24492,#24493,#24494,#24495,#24496,#24497,#24498,#24499,
#24500,#24501,#24502,#24503,#24504,#24505,#24506,#24507,#24508,#24509,#24510,
#24511,#24512,#24513,#24514,#24515,#24516,#24517,#24518,#24519,#24520,#24521,
#24522,#24523,#24524,#24525,#24526,#24527,#24528,#24529,#24530,#24531,#24532,
#24533,#24534,#24535,#24536,#24537,#24538,#24539,#24540,#24541,#24542,#24543,
#24544,#24545,#24546,#24547,#24548,#24549,#24550,#24551,#24552,#24553),
 .UNSPECIFIED.,.F.,.F.,(4,3,3,3,3,3,3,3,3,3,3,3,3,3,3,3,3,3,3,3,3,3,3,4),
(0.,0.079016546580938,0.157641122394585,0.183993443720854,0.207891281656444,
0.251131687956984,0.328243571587973,0.374168384090539,0.397099877179475,
0.472026294619315,0.492301725366521,0.550056206928688,0.568103933485432,
0.584735378149958,0.65759847554391,0.72331965161519,0.743939980328521,0.763679188248337,
0.809798919188833,0.846311488438111,0.867561854219163,0.937273050771799,
0.943726018375008,0.954382097139032),.UNSPECIFIED.);
#2272=B_SPLINE_CURVE_WITH_KNOTS('',3,(#24569,#24570,#24571,#24572,#24573,
#24574,#24575,#24576,#24577,#24578,#24579,#24580,#24581,#24582,#24583,#24584,
#24585,#24586),.UNSPECIFIED.,.F.,.F.,(4,2,2,2,2,2,2,2,4),(0.,0.0759876362447371,
0.151975272489474,0.227927665609885,0.303880058730296,0.379832451850707,
0.455784844971118,0.531772481215855,0.607760117460592),.UNSPECIFIED.);
#2273=B_SPLINE_CURVE_WITH_KNOTS('',3,(#24587,#24588,#24589,#24590,#24591,
#24592,#24593,#24594,#24595,#24596,#24597,#24598,#24599,#24600,#24601,#24602,
#24603,#24604),.UNSPECIFIED.,.F.,.F.,(4,2,2,2,2,2,2,2,4),(0.607760117460592,
0.68374775370533,0.759735389950067,0.835687783070478,0.911640176190889,
0.9875925693113,1.06354496243171,1.13953259867645,1.21552023492118),
 .UNSPECIFIED.);
#2274=B_SPLINE_CURVE_WITH_KNOTS('',3,(#24609,#24610,#24611,#24612,#24613,
#24614,#24615,#24616,#24617,#24618,#24619,#24620,#24621),.UNSPECIFIED.,
 .F.,.F.,(4,2,3,2,2,4),(-0.408608378270607,-0.265388212066323,0.,0.265388212066323,
0.530776424132647,0.698056008856335),.UNSPECIFIED.);
#2275=B_SPLINE_CURVE_WITH_KNOTS('',3,(#24624,#24625,#24626,#24627,#24628,
#24629,#24630,#24631,#24632,#24633,#24634,#24635),.UNSPECIFIED.,.F.,.F.,
(4,2,2,2,2,4),(1.42476853019388,1.59204811491757,1.85743632698389,2.12282453905022,
2.38821275111654,2.53143291732083),.UNSPECIFIED.);
#2276=B_SPLINE_CURVE_WITH_KNOTS('',3,(#24669,#24670,#24671,#24672,#24673,
#24674,#24675,#24676,#24677,#24678,#24679,#24680,#24681),.UNSPECIFIED.,
 .F.,.F.,(4,2,3,2,2,4),(-0.408608378270607,-0.265388212066323,0.,0.265388212066323,
0.530776424132647,0.698056008856335),.UNSPECIFIED.);
#2277=B_SPLINE_CURVE_WITH_KNOTS('',3,(#24697,#24698,#24699,#24700,#24701,
#24702,#24703,#24704,#24705,#24706),.UNSPECIFIED.,.F.,.F.,(4,2,2,2,4),(0.303880058730296,
0.379832451850707,0.455784844971118,0.531772481215855,0.607760117460592),
 .UNSPECIFIED.);
#2278=B_SPLINE_CURVE_WITH_KNOTS('',3,(#24708,#24709,#24710,#24711,#24712,
#24713,#24714,#24715,#24716,#24717),.UNSPECIFIED.,.F.,.F.,(4,2,2,2,4),(0.,
0.0759876362447371,0.151975272489474,0.227927665609885,0.303880058730296),
 .UNSPECIFIED.);
#2279=B_SPLINE_CURVE_WITH_KNOTS('',3,(#24719,#24720,#24721,#24722,#24723,
#24724,#24725,#24726,#24727,#24728),.UNSPECIFIED.,.F.,.F.,(4,2,2,2,4),(0.911640176190889,
0.9875925693113,1.06354496243171,1.13953259867645,1.21552023492118),
 .UNSPECIFIED.);
#2280=B_SPLINE_CURVE_WITH_KNOTS('',3,(#24729,#24730,#24731,#24732,#24733,
#24734,#24735,#24736,#24737,#24738),.UNSPECIFIED.,.F.,.F.,(4,2,2,2,4),(0.607760117460592,
0.68374775370533,0.759735389950067,0.835687783070478,0.911640176190889),
 .UNSPECIFIED.);
#2281=B_SPLINE_CURVE_WITH_KNOTS('',3,(#24742,#24743,#24744,#24745,#24746,
#24747,#24748,#24749,#24750,#24751,#24752,#24753),.UNSPECIFIED.,.F.,.F.,
(4,2,2,2,2,4),(1.42476853019388,1.59204811491757,1.85743632698389,2.12282453905022,
2.38821275111654,2.53143291732083),.UNSPECIFIED.);
#2995=LINE('',#22264,#3627);
#2996=LINE('',#22321,#3628);
#2997=LINE('',#22408,#3629);
#2998=LINE('',#22477,#3630);
#2999=LINE('',#22534,#3631);
#3000=LINE('',#22621,#3632);
#3001=LINE('',#22690,#3633);
#3002=LINE('',#22706,#3634);
#3003=LINE('',#22744,#3635);
#3004=LINE('',#22780,#3636);
#3005=LINE('',#22800,#3637);
#3006=LINE('',#22816,#3638);
#3007=LINE('',#22854,#3639);
#3008=LINE('',#22890,#3640);
#3009=LINE('',#22912,#3641);
#3010=LINE('',#22913,#3642);
#3011=LINE('',#22919,#3643);
#3012=LINE('',#22920,#3644);
#3013=LINE('',#22924,#3645);
#3014=LINE('',#22926,#3646);
#3015=LINE('',#22928,#3647);
#3016=LINE('',#22929,#3648);
#3017=LINE('',#22933,#3649);
#3018=LINE('',#22935,#3650);
#3019=LINE('',#22937,#3651);
#3020=LINE('',#22938,#3652);
#3021=LINE('',#22942,#3653);
#3022=LINE('',#22945,#3654);
#3023=LINE('',#22947,#3655);
#3024=LINE('',#22948,#3656);
#3025=LINE('',#22951,#3657);
#3026=LINE('',#22953,#3658);
#3027=LINE('',#22954,#3659);
#3028=LINE('',#22958,#3660);
#3029=LINE('',#22960,#3661);
#3030=LINE('',#22962,#3662);
#3031=LINE('',#24560,#3663);
#3032=LINE('',#24567,#3664);
#3033=LINE('',#24608,#3665);
#3034=LINE('',#24637,#3666);
#3035=LINE('',#24641,#3667);
#3036=LINE('',#24645,#3668);
#3037=LINE('',#24647,#3669);
#3038=LINE('',#24649,#3670);
#3039=LINE('',#24650,#3671);
#3040=LINE('',#24662,#3672);
#3041=LINE('',#24664,#3673);
#3042=LINE('',#24666,#3674);
#3043=LINE('',#24688,#3675);
#3044=LINE('',#24695,#3676);
#3045=LINE('',#24757,#3677);
#3046=LINE('',#24761,#3678);
#3047=LINE('',#24765,#3679);
#3048=LINE('',#24769,#3680);
#3049=LINE('',#24772,#3681);
#3050=LINE('',#24774,#3682);
#3051=LINE('',#24779,#3683);
#3052=LINE('',#24780,#3684);
#3053=LINE('',#24781,#3685);
#3054=LINE('',#24784,#3686);
#3055=LINE('',#24785,#3687);
#3056=LINE('',#24788,#3688);
#3057=LINE('',#24789,#3689);
#3058=LINE('',#24791,#3690);
#3627=VECTOR('',#12836,0.5);
#3628=VECTOR('',#12841,0.5);
#3629=VECTOR('',#12844,0.5);
#3630=VECTOR('',#12849,0.5);
#3631=VECTOR('',#12854,0.5);
#3632=VECTOR('',#12857,0.5);
#3633=VECTOR('',#12862,0.5099);
#3634=VECTOR('',#12867,0.5099);
#3635=VECTOR('',#12870,0.5099);
#3636=VECTOR('',#12873,0.5099);
#3637=VECTOR('',#12878,0.5099);
#3638=VECTOR('',#12883,0.5099);
#3639=VECTOR('',#12886,0.5099);
#3640=VECTOR('',#12889,0.5099);
#3641=VECTOR('',#12896,1.);
#3642=VECTOR('',#12897,1.);
#3643=VECTOR('',#12902,1.);
#3644=VECTOR('',#12903,1.);
#3645=VECTOR('',#12906,1.);
#3646=VECTOR('',#12907,1.);
#3647=VECTOR('',#12908,1.);
#3648=VECTOR('',#12909,1.);
#3649=VECTOR('',#12912,1.);
#3650=VECTOR('',#12913,1.);
#3651=VECTOR('',#12914,1.);
#3652=VECTOR('',#12915,1.);
#3653=VECTOR('',#12920,1.);
#3654=VECTOR('',#12923,1.);
#3655=VECTOR('',#12924,1.);
#3656=VECTOR('',#12925,1.);
#3657=VECTOR('',#12928,1.);
#3658=VECTOR('',#12929,1.);
#3659=VECTOR('',#12930,1.);
#3660=VECTOR('',#12935,1.);
#3661=VECTOR('',#12938,1.);
#3662=VECTOR('',#12941,1.);
#3663=VECTOR('',#12962,0.4);
#3664=VECTOR('',#12971,0.2);
#3665=VECTOR('',#12974,1.);
#3666=VECTOR('',#12977,1.);
#3667=VECTOR('',#12984,1.);
#3668=VECTOR('',#12987,1.);
#3669=VECTOR('',#12988,1.);
#3670=VECTOR('',#12989,1.);
#3671=VECTOR('',#12990,1.);
#3672=VECTOR('',#13001,1.);
#3673=VECTOR('',#13002,1.);
#3674=VECTOR('',#13003,1.);
#3675=VECTOR('',#13016,0.4);
#3676=VECTOR('',#13025,0.2);
#3677=VECTOR('',#13036,0.25);
#3678=VECTOR('',#13041,0.25);
#3679=VECTOR('',#13046,0.25);
#3680=VECTOR('',#13051,0.25);
#3681=VECTOR('',#13056,0.6);
#3682=VECTOR('',#13057,0.6);
#3683=VECTOR('',#13062,1.);
#3684=VECTOR('',#13063,1.);
#3685=VECTOR('',#13064,1.);
#3686=VECTOR('',#13067,1.);
#3687=VECTOR('',#13068,1.);
#3688=VECTOR('',#13071,1.);
#3689=VECTOR('',#13072,1.);
#3690=VECTOR('',#13075,1.);
#4392=VERTEX_POINT('',#22262);
#4393=VERTEX_POINT('',#22263);
#4394=VERTEX_POINT('',#22265);
#4395=VERTEX_POINT('',#22285);
#4396=VERTEX_POINT('',#22319);
#4397=VERTEX_POINT('',#22320);
#4398=VERTEX_POINT('',#22406);
#4399=VERTEX_POINT('',#22407);
#4400=VERTEX_POINT('',#22409);
#4401=VERTEX_POINT('',#22435);
#4402=VERTEX_POINT('',#22475);
#4403=VERTEX_POINT('',#22476);
#4404=VERTEX_POINT('',#22478);
#4405=VERTEX_POINT('',#22498);
#4406=VERTEX_POINT('',#22532);
#4407=VERTEX_POINT('',#22533);
#4408=VERTEX_POINT('',#22619);
#4409=VERTEX_POINT('',#22620);
#4410=VERTEX_POINT('',#22622);
#4411=VERTEX_POINT('',#22648);
#4412=VERTEX_POINT('',#22688);
#4413=VERTEX_POINT('',#22689);
#4414=VERTEX_POINT('',#22691);
#4415=VERTEX_POINT('',#22696);
#4416=VERTEX_POINT('',#22704);
#4417=VERTEX_POINT('',#22705);
#4418=VERTEX_POINT('',#22742);
#4419=VERTEX_POINT('',#22743);
#4420=VERTEX_POINT('',#22778);
#4421=VERTEX_POINT('',#22779);
#4422=VERTEX_POINT('',#22781);
#4423=VERTEX_POINT('',#22788);
#4424=VERTEX_POINT('',#22798);
#4425=VERTEX_POINT('',#22799);
#4426=VERTEX_POINT('',#22801);
#4427=VERTEX_POINT('',#22806);
#4428=VERTEX_POINT('',#22814);
#4429=VERTEX_POINT('',#22815);
#4430=VERTEX_POINT('',#22852);
#4431=VERTEX_POINT('',#22853);
#4432=VERTEX_POINT('',#22888);
#4433=VERTEX_POINT('',#22889);
#4434=VERTEX_POINT('',#22891);
#4435=VERTEX_POINT('',#22898);
#4436=VERTEX_POINT('',#22908);
#4437=VERTEX_POINT('',#22909);
#4438=VERTEX_POINT('',#22911);
#4439=VERTEX_POINT('',#22915);
#4440=VERTEX_POINT('',#22916);
#4441=VERTEX_POINT('',#22918);
#4442=VERTEX_POINT('',#22922);
#4443=VERTEX_POINT('',#22923);
#4444=VERTEX_POINT('',#22925);
#4445=VERTEX_POINT('',#22927);
#4446=VERTEX_POINT('',#22931);
#4447=VERTEX_POINT('',#22932);
#4448=VERTEX_POINT('',#22934);
#4449=VERTEX_POINT('',#22936);
#4450=VERTEX_POINT('',#22940);
#4451=VERTEX_POINT('',#22944);
#4452=VERTEX_POINT('',#22946);
#4453=VERTEX_POINT('',#22950);
#4454=VERTEX_POINT('',#22952);
#4455=VERTEX_POINT('',#22956);
#4456=VERTEX_POINT('',#22964);
#4457=VERTEX_POINT('',#24556);
#4458=VERTEX_POINT('',#24559);
#4459=VERTEX_POINT('',#24563);
#4460=VERTEX_POINT('',#24566);
#4461=VERTEX_POINT('',#24568);
#4462=VERTEX_POINT('',#24606);
#4463=VERTEX_POINT('',#24607);
#4464=VERTEX_POINT('',#24623);
#4465=VERTEX_POINT('',#24636);
#4466=VERTEX_POINT('',#24643);
#4467=VERTEX_POINT('',#24644);
#4468=VERTEX_POINT('',#24646);
#4469=VERTEX_POINT('',#24648);
#4470=VERTEX_POINT('',#24651);
#4471=VERTEX_POINT('',#24653);
#4472=VERTEX_POINT('',#24655);
#4473=VERTEX_POINT('',#24657);
#4474=VERTEX_POINT('',#24659);
#4475=VERTEX_POINT('',#24661);
#4476=VERTEX_POINT('',#24663);
#4477=VERTEX_POINT('',#24665);
#4478=VERTEX_POINT('',#24684);
#4479=VERTEX_POINT('',#24687);
#4480=VERTEX_POINT('',#24691);
#4481=VERTEX_POINT('',#24694);
#4482=VERTEX_POINT('',#24696);
#4483=VERTEX_POINT('',#24707);
#4484=VERTEX_POINT('',#24718);
#4485=VERTEX_POINT('',#24756);
#4486=VERTEX_POINT('',#24760);
#4487=VERTEX_POINT('',#24764);
#4488=VERTEX_POINT('',#24768);
#4489=VERTEX_POINT('',#24773);
#4490=VERTEX_POINT('',#24777);
#4491=VERTEX_POINT('',#24778);
#4492=VERTEX_POINT('',#24783);
#4493=VERTEX_POINT('',#24787);
#5647=EDGE_CURVE('',#4392,#4393,#2995,.T.);
#5648=EDGE_CURVE('',#4393,#4394,#2228,.T.);
#5649=EDGE_CURVE('',#4394,#4395,#1847,.F.);
#5650=EDGE_CURVE('',#4395,#4392,#2229,.T.);
#5651=EDGE_CURVE('',#4396,#4397,#2996,.T.);
#5652=EDGE_CURVE('',#4397,#4393,#2230,.T.);
#5653=EDGE_CURVE('',#4392,#4396,#2231,.T.);
#5654=EDGE_CURVE('',#4398,#4399,#2997,.T.);
#5655=EDGE_CURVE('',#4398,#4400,#2232,.T.);
#5656=EDGE_CURVE('',#4401,#4400,#1848,.F.);
#5657=EDGE_CURVE('',#4401,#4399,#2233,.T.);
#5658=EDGE_CURVE('',#4402,#4403,#2998,.T.);
#5659=EDGE_CURVE('',#4403,#4404,#2234,.T.);
#5660=EDGE_CURVE('',#4404,#4405,#1849,.F.);
#5661=EDGE_CURVE('',#4405,#4402,#2235,.T.);
#5662=EDGE_CURVE('',#4406,#4407,#2999,.T.);
#5663=EDGE_CURVE('',#4407,#4403,#2236,.T.);
#5664=EDGE_CURVE('',#4402,#4406,#2237,.T.);
#5665=EDGE_CURVE('',#4408,#4409,#3000,.T.);
#5666=EDGE_CURVE('',#4408,#4410,#2238,.T.);
#5667=EDGE_CURVE('',#4411,#4410,#1850,.T.);
#5668=EDGE_CURVE('',#4411,#4409,#2239,.T.);
#5669=EDGE_CURVE('',#4412,#4413,#3001,.T.);
#5670=EDGE_CURVE('',#4413,#4414,#2240,.T.);
#5671=EDGE_CURVE('',#4415,#4414,#1851,.T.);
#5672=EDGE_CURVE('',#4412,#4415,#2241,.T.);
#5673=EDGE_CURVE('',#4416,#4417,#3002,.T.);
#5674=EDGE_CURVE('',#4417,#4413,#2242,.T.);
#5675=EDGE_CURVE('',#4416,#4412,#2243,.T.);
#5676=EDGE_CURVE('',#4418,#4419,#3003,.T.);
#5677=EDGE_CURVE('',#4419,#4417,#2244,.T.);
#5678=EDGE_CURVE('',#4418,#4416,#2245,.T.);
#5679=EDGE_CURVE('',#4420,#4421,#3004,.T.);
#5680=EDGE_CURVE('',#4422,#4420,#2246,.T.);
#5681=EDGE_CURVE('',#4423,#4422,#1852,.T.);
#5682=EDGE_CURVE('',#4423,#4421,#2247,.T.);
#5683=EDGE_CURVE('',#4424,#4425,#3005,.T.);
#5684=EDGE_CURVE('',#4425,#4426,#2248,.T.);
#5685=EDGE_CURVE('',#4427,#4426,#1853,.T.);
#5686=EDGE_CURVE('',#4424,#4427,#2249,.T.);
#5687=EDGE_CURVE('',#4428,#4429,#3006,.T.);
#5688=EDGE_CURVE('',#4429,#4425,#2250,.T.);
#5689=EDGE_CURVE('',#4428,#4424,#2251,.T.);
#5690=EDGE_CURVE('',#4430,#4431,#3007,.T.);
#5691=EDGE_CURVE('',#4431,#4429,#2252,.T.);
#5692=EDGE_CURVE('',#4430,#4428,#2253,.T.);
#5693=EDGE_CURVE('',#4432,#4433,#3008,.T.);
#5694=EDGE_CURVE('',#4434,#4432,#2254,.T.);
#5695=EDGE_CURVE('',#4435,#4434,#1854,.T.);
#5696=EDGE_CURVE('',#4435,#4433,#2255,.T.);
#5697=EDGE_CURVE('',#4436,#4437,#1855,.T.);
#5698=EDGE_CURVE('',#4436,#4438,#3009,.T.);
#5699=EDGE_CURVE('',#4437,#4438,#3010,.T.);
#5700=EDGE_CURVE('',#4439,#4440,#1856,.T.);
#5701=EDGE_CURVE('',#4441,#4440,#3011,.T.);
#5702=EDGE_CURVE('',#4439,#4441,#3012,.T.);
#5703=EDGE_CURVE('',#4442,#4443,#3013,.T.);
#5704=EDGE_CURVE('',#4443,#4444,#3014,.T.);
#5705=EDGE_CURVE('',#4445,#4444,#3015,.T.);
#5706=EDGE_CURVE('',#4442,#4445,#3016,.T.);
#5707=EDGE_CURVE('',#4446,#4447,#3017,.T.);
#5708=EDGE_CURVE('',#4447,#4448,#3018,.T.);
#5709=EDGE_CURVE('',#4449,#4448,#3019,.T.);
#5710=EDGE_CURVE('',#4446,#4449,#3020,.T.);
#5711=EDGE_CURVE('',#4450,#4446,#1857,.T.);
#5712=EDGE_CURVE('',#4450,#4449,#3021,.T.);
#5713=EDGE_CURVE('',#4451,#4439,#3022,.T.);
#5714=EDGE_CURVE('',#4452,#4441,#3023,.T.);
#5715=EDGE_CURVE('',#4451,#4452,#3024,.T.);
#5716=EDGE_CURVE('',#4436,#4453,#3025,.T.);
#5717=EDGE_CURVE('',#4453,#4454,#3026,.T.);
#5718=EDGE_CURVE('',#4438,#4454,#3027,.T.);
#5719=EDGE_CURVE('',#4455,#4443,#1858,.T.);
#5720=EDGE_CURVE('',#4444,#4455,#3028,.T.);
#5721=EDGE_CURVE('',#4437,#4455,#3029,.T.);
#5722=EDGE_CURVE('',#4454,#4452,#1859,.T.);
#5723=EDGE_CURVE('',#4450,#4440,#3030,.T.);
#5724=EDGE_CURVE('',#4448,#4445,#1860,.T.);
#5725=EDGE_CURVE('',#4456,#4456,#1861,.T.);
#5726=EDGE_CURVE('',#4440,#4450,#1862,.T.);
#5727=EDGE_CURVE('',#4433,#4431,#2256,.T.);
#5728=EDGE_CURVE('',#4432,#4430,#2257,.T.);
#5729=EDGE_CURVE('',#4426,#4405,#2258,.T.);
#5730=EDGE_CURVE('',#4410,#4435,#2259,.T.);
#5731=EDGE_CURVE('',#4406,#4408,#2260,.T.);
#5732=EDGE_CURVE('',#4404,#4427,#2261,.T.);
#5733=EDGE_CURVE('',#4409,#4407,#2262,.T.);
#5734=EDGE_CURVE('',#4434,#4411,#2263,.T.);
#5735=EDGE_CURVE('',#4421,#4419,#2264,.T.);
#5736=EDGE_CURVE('',#4420,#4418,#2265,.T.);
#5737=EDGE_CURVE('',#4414,#4395,#2266,.T.);
#5738=EDGE_CURVE('',#4400,#4423,#2267,.T.);
#5739=EDGE_CURVE('',#4396,#4398,#2268,.T.);
#5740=EDGE_CURVE('',#4394,#4415,#2269,.T.);
#5741=EDGE_CURVE('',#4399,#4397,#2270,.T.);
#5742=EDGE_CURVE('',#4422,#4401,#2271,.T.);
#5743=EDGE_CURVE('',#4457,#4457,#1863,.T.);
#5744=EDGE_CURVE('',#4457,#4458,#3031,.T.);
#5745=EDGE_CURVE('',#4458,#4458,#1864,.T.);
#5746=EDGE_CURVE('',#4459,#4459,#1865,.T.);
#5747=EDGE_CURVE('',#4459,#4460,#3032,.T.);
#5748=EDGE_CURVE('',#4461,#4460,#2272,.T.);
#5749=EDGE_CURVE('',#4460,#4461,#2273,.T.);
#5750=EDGE_CURVE('',#4462,#4463,#3033,.T.);
#5751=EDGE_CURVE('',#4453,#4462,#2274,.T.);
#5752=EDGE_CURVE('',#4437,#4455,#1866,.T.);
#5753=EDGE_CURVE('',#4464,#4442,#2275,.T.);
#5754=EDGE_CURVE('',#4465,#4464,#3034,.T.);
#5755=EDGE_CURVE('',#4463,#4465,#1867,.T.);
#5756=EDGE_CURVE('',#4463,#4465,#3035,.T.);
#5757=EDGE_CURVE('',#4466,#4467,#3036,.T.);
#5758=EDGE_CURVE('',#4467,#4468,#3037,.T.);
#5759=EDGE_CURVE('',#4468,#4469,#3038,.T.);
#5760=EDGE_CURVE('',#4469,#4466,#3039,.T.);
#5761=EDGE_CURVE('',#4470,#4470,#1868,.T.);
#5762=EDGE_CURVE('',#4471,#4471,#1869,.T.);
#5763=EDGE_CURVE('',#4472,#4472,#1870,.T.);
#5764=EDGE_CURVE('',#4473,#4473,#1871,.T.);
#5765=EDGE_CURVE('',#4464,#4474,#1872,.T.);
#5766=EDGE_CURVE('',#4474,#4475,#3040,.T.);
#5767=EDGE_CURVE('',#4475,#4476,#3041,.T.);
#5768=EDGE_CURVE('',#4476,#4477,#3042,.T.);
#5769=EDGE_CURVE('',#4477,#4462,#1873,.T.);
#5770=EDGE_CURVE('',#4447,#4474,#2276,.T.);
#5771=EDGE_CURVE('',#4478,#4478,#1874,.T.);
#5772=EDGE_CURVE('',#4478,#4479,#3043,.T.);
#5773=EDGE_CURVE('',#4479,#4479,#1875,.T.);
#5774=EDGE_CURVE('',#4480,#4480,#1876,.T.);
#5775=EDGE_CURVE('',#4480,#4481,#3044,.T.);
#5776=EDGE_CURVE('',#4482,#4481,#2277,.T.);
#5777=EDGE_CURVE('',#4483,#4482,#2278,.T.);
#5778=EDGE_CURVE('',#4484,#4483,#2279,.T.);
#5779=EDGE_CURVE('',#4481,#4484,#2280,.T.);
#5780=EDGE_CURVE('',#4475,#4476,#1877,.T.);
#5781=EDGE_CURVE('',#4477,#4451,#2281,.T.);
#5782=EDGE_CURVE('',#4470,#4485,#3045,.T.);
#5783=EDGE_CURVE('',#4485,#4485,#1878,.T.);
#5784=EDGE_CURVE('',#4471,#4486,#3046,.T.);
#5785=EDGE_CURVE('',#4486,#4486,#1879,.T.);
#5786=EDGE_CURVE('',#4472,#4487,#3047,.T.);
#5787=EDGE_CURVE('',#4487,#4487,#1880,.T.);
#5788=EDGE_CURVE('',#4473,#4488,#3048,.T.);
#5789=EDGE_CURVE('',#4488,#4488,#1881,.T.);
#5790=EDGE_CURVE('',#4456,#4482,#3049,.T.);
#5791=EDGE_CURVE('',#4484,#4489,#3050,.T.);
#5792=EDGE_CURVE('',#4489,#4489,#1882,.T.);
#5793=EDGE_CURVE('',#4490,#4491,#3051,.T.);
#5794=EDGE_CURVE('',#4491,#4466,#3052,.T.);
#5795=EDGE_CURVE('',#4490,#4469,#3053,.T.);
#5796=EDGE_CURVE('',#4492,#4490,#3054,.T.);
#5797=EDGE_CURVE('',#4492,#4468,#3055,.T.);
#5798=EDGE_CURVE('',#4493,#4492,#3056,.T.);
#5799=EDGE_CURVE('',#4493,#4467,#3057,.T.);
#5800=EDGE_CURVE('',#4491,#4493,#3058,.T.);
#7755=ORIENTED_EDGE('',*,*,#5647,.T.);
#7756=ORIENTED_EDGE('',*,*,#5648,.T.);
#7757=ORIENTED_EDGE('',*,*,#5649,.T.);
#7758=ORIENTED_EDGE('',*,*,#5650,.T.);
#7759=ORIENTED_EDGE('',*,*,#5651,.T.);
#7760=ORIENTED_EDGE('',*,*,#5652,.T.);
#7761=ORIENTED_EDGE('',*,*,#5647,.F.);
#7762=ORIENTED_EDGE('',*,*,#5653,.T.);
#7763=ORIENTED_EDGE('',*,*,#5654,.F.);
#7764=ORIENTED_EDGE('',*,*,#5655,.T.);
#7765=ORIENTED_EDGE('',*,*,#5656,.F.);
#7766=ORIENTED_EDGE('',*,*,#5657,.T.);
#7767=ORIENTED_EDGE('',*,*,#5658,.T.);
#7768=ORIENTED_EDGE('',*,*,#5659,.T.);
#7769=ORIENTED_EDGE('',*,*,#5660,.T.);
#7770=ORIENTED_EDGE('',*,*,#5661,.T.);
#7771=ORIENTED_EDGE('',*,*,#5662,.T.);
#7772=ORIENTED_EDGE('',*,*,#5663,.T.);
#7773=ORIENTED_EDGE('',*,*,#5658,.F.);
#7774=ORIENTED_EDGE('',*,*,#5664,.T.);
#7775=ORIENTED_EDGE('',*,*,#5665,.F.);
#7776=ORIENTED_EDGE('',*,*,#5666,.T.);
#7777=ORIENTED_EDGE('',*,*,#5667,.F.);
#7778=ORIENTED_EDGE('',*,*,#5668,.T.);
#7779=ORIENTED_EDGE('',*,*,#5669,.T.);
#7780=ORIENTED_EDGE('',*,*,#5670,.T.);
#7781=ORIENTED_EDGE('',*,*,#5671,.F.);
#7782=ORIENTED_EDGE('',*,*,#5672,.F.);
#7783=ORIENTED_EDGE('',*,*,#5673,.T.);
#7784=ORIENTED_EDGE('',*,*,#5674,.T.);
#7785=ORIENTED_EDGE('',*,*,#5669,.F.);
#7786=ORIENTED_EDGE('',*,*,#5675,.F.);
#7787=ORIENTED_EDGE('',*,*,#5676,.T.);
#7788=ORIENTED_EDGE('',*,*,#5677,.T.);
#7789=ORIENTED_EDGE('',*,*,#5673,.F.);
#7790=ORIENTED_EDGE('',*,*,#5678,.F.);
#7791=ORIENTED_EDGE('',*,*,#5679,.F.);
#7792=ORIENTED_EDGE('',*,*,#5680,.F.);
#7793=ORIENTED_EDGE('',*,*,#5681,.F.);
#7794=ORIENTED_EDGE('',*,*,#5682,.T.);
#7795=ORIENTED_EDGE('',*,*,#5683,.T.);
#7796=ORIENTED_EDGE('',*,*,#5684,.T.);
#7797=ORIENTED_EDGE('',*,*,#5685,.F.);
#7798=ORIENTED_EDGE('',*,*,#5686,.F.);
#7799=ORIENTED_EDGE('',*,*,#5687,.T.);
#7800=ORIENTED_EDGE('',*,*,#5688,.T.);
#7801=ORIENTED_EDGE('',*,*,#5683,.F.);
#7802=ORIENTED_EDGE('',*,*,#5689,.F.);
#7803=ORIENTED_EDGE('',*,*,#5690,.T.);
#7804=ORIENTED_EDGE('',*,*,#5691,.T.);
#7805=ORIENTED_EDGE('',*,*,#5687,.F.);
#7806=ORIENTED_EDGE('',*,*,#5692,.F.);
#7807=ORIENTED_EDGE('',*,*,#5693,.F.);
#7808=ORIENTED_EDGE('',*,*,#5694,.F.);
#7809=ORIENTED_EDGE('',*,*,#5695,.F.);
#7810=ORIENTED_EDGE('',*,*,#5696,.T.);
#7811=ORIENTED_EDGE('',*,*,#5697,.F.);
#7812=ORIENTED_EDGE('',*,*,#5698,.T.);
#7813=ORIENTED_EDGE('',*,*,#5699,.F.);
#7814=ORIENTED_EDGE('',*,*,#5700,.T.);
#7815=ORIENTED_EDGE('',*,*,#5701,.F.);
#7816=ORIENTED_EDGE('',*,*,#5702,.F.);
#7817=ORIENTED_EDGE('',*,*,#5703,.T.);
#7818=ORIENTED_EDGE('',*,*,#5704,.T.);
#7819=ORIENTED_EDGE('',*,*,#5705,.F.);
#7820=ORIENTED_EDGE('',*,*,#5706,.F.);
#7821=ORIENTED_EDGE('',*,*,#5707,.T.);
#7822=ORIENTED_EDGE('',*,*,#5708,.T.);
#7823=ORIENTED_EDGE('',*,*,#5709,.F.);
#7824=ORIENTED_EDGE('',*,*,#5710,.F.);
#7825=ORIENTED_EDGE('',*,*,#5711,.T.);
#7826=ORIENTED_EDGE('',*,*,#5710,.T.);
#7827=ORIENTED_EDGE('',*,*,#5712,.F.);
#7828=ORIENTED_EDGE('',*,*,#5713,.T.);
#7829=ORIENTED_EDGE('',*,*,#5702,.T.);
#7830=ORIENTED_EDGE('',*,*,#5714,.F.);
#7831=ORIENTED_EDGE('',*,*,#5715,.F.);
#7832=ORIENTED_EDGE('',*,*,#5716,.T.);
#7833=ORIENTED_EDGE('',*,*,#5717,.T.);
#7834=ORIENTED_EDGE('',*,*,#5718,.F.);
#7835=ORIENTED_EDGE('',*,*,#5698,.F.);
#7836=ORIENTED_EDGE('',*,*,#5719,.F.);
#7837=ORIENTED_EDGE('',*,*,#5720,.F.);
#7838=ORIENTED_EDGE('',*,*,#5704,.F.);
#7839=ORIENTED_EDGE('',*,*,#5720,.T.);
#7840=ORIENTED_EDGE('',*,*,#5721,.F.);
#7841=ORIENTED_EDGE('',*,*,#5699,.T.);
#7842=ORIENTED_EDGE('',*,*,#5718,.T.);
#7843=ORIENTED_EDGE('',*,*,#5722,.T.);
#7844=ORIENTED_EDGE('',*,*,#5714,.T.);
#7845=ORIENTED_EDGE('',*,*,#5701,.T.);
#7846=ORIENTED_EDGE('',*,*,#5723,.F.);
#7847=ORIENTED_EDGE('',*,*,#5712,.T.);
#7848=ORIENTED_EDGE('',*,*,#5709,.T.);
#7849=ORIENTED_EDGE('',*,*,#5724,.T.);
#7850=ORIENTED_EDGE('',*,*,#5705,.T.);
#7851=ORIENTED_EDGE('',*,*,#5725,.T.);
#7852=ORIENTED_EDGE('',*,*,#5723,.T.);
#7853=ORIENTED_EDGE('',*,*,#5726,.T.);
#7854=ORIENTED_EDGE('',*,*,#5693,.T.);
#7855=ORIENTED_EDGE('',*,*,#5727,.T.);
#7856=ORIENTED_EDGE('',*,*,#5690,.F.);
#7857=ORIENTED_EDGE('',*,*,#5728,.F.);
#7858=ORIENTED_EDGE('',*,*,#5729,.F.);
#7859=ORIENTED_EDGE('',*,*,#5684,.F.);
#7860=ORIENTED_EDGE('',*,*,#5688,.F.);
#7861=ORIENTED_EDGE('',*,*,#5691,.F.);
#7862=ORIENTED_EDGE('',*,*,#5727,.F.);
#7863=ORIENTED_EDGE('',*,*,#5696,.F.);
#7864=ORIENTED_EDGE('',*,*,#5730,.F.);
#7865=ORIENTED_EDGE('',*,*,#5666,.F.);
#7866=ORIENTED_EDGE('',*,*,#5731,.F.);
#7867=ORIENTED_EDGE('',*,*,#5664,.F.);
#7868=ORIENTED_EDGE('',*,*,#5661,.F.);
#7869=ORIENTED_EDGE('',*,*,#5732,.F.);
#7870=ORIENTED_EDGE('',*,*,#5659,.F.);
#7871=ORIENTED_EDGE('',*,*,#5663,.F.);
#7872=ORIENTED_EDGE('',*,*,#5733,.F.);
#7873=ORIENTED_EDGE('',*,*,#5668,.F.);
#7874=ORIENTED_EDGE('',*,*,#5734,.F.);
#7875=ORIENTED_EDGE('',*,*,#5694,.T.);
#7876=ORIENTED_EDGE('',*,*,#5728,.T.);
#7877=ORIENTED_EDGE('',*,*,#5692,.T.);
#7878=ORIENTED_EDGE('',*,*,#5689,.T.);
#7879=ORIENTED_EDGE('',*,*,#5686,.T.);
#7880=ORIENTED_EDGE('',*,*,#5679,.T.);
#7881=ORIENTED_EDGE('',*,*,#5735,.T.);
#7882=ORIENTED_EDGE('',*,*,#5676,.F.);
#7883=ORIENTED_EDGE('',*,*,#5736,.F.);
#7884=ORIENTED_EDGE('',*,*,#5737,.F.);
#7885=ORIENTED_EDGE('',*,*,#5670,.F.);
#7886=ORIENTED_EDGE('',*,*,#5674,.F.);
#7887=ORIENTED_EDGE('',*,*,#5677,.F.);
#7888=ORIENTED_EDGE('',*,*,#5735,.F.);
#7889=ORIENTED_EDGE('',*,*,#5682,.F.);
#7890=ORIENTED_EDGE('',*,*,#5738,.F.);
#7891=ORIENTED_EDGE('',*,*,#5655,.F.);
#7892=ORIENTED_EDGE('',*,*,#5739,.F.);
#7893=ORIENTED_EDGE('',*,*,#5653,.F.);
#7894=ORIENTED_EDGE('',*,*,#5650,.F.);
#7895=ORIENTED_EDGE('',*,*,#5740,.F.);
#7896=ORIENTED_EDGE('',*,*,#5648,.F.);
#7897=ORIENTED_EDGE('',*,*,#5652,.F.);
#7898=ORIENTED_EDGE('',*,*,#5741,.F.);
#7899=ORIENTED_EDGE('',*,*,#5657,.F.);
#7900=ORIENTED_EDGE('',*,*,#5742,.F.);
#7901=ORIENTED_EDGE('',*,*,#5680,.T.);
#7902=ORIENTED_EDGE('',*,*,#5736,.T.);
#7903=ORIENTED_EDGE('',*,*,#5678,.T.);
#7904=ORIENTED_EDGE('',*,*,#5675,.T.);
#7905=ORIENTED_EDGE('',*,*,#5672,.T.);
#7906=ORIENTED_EDGE('',*,*,#5665,.T.);
#7907=ORIENTED_EDGE('',*,*,#5733,.T.);
#7908=ORIENTED_EDGE('',*,*,#5662,.F.);
#7909=ORIENTED_EDGE('',*,*,#5731,.T.);
#7910=ORIENTED_EDGE('',*,*,#5732,.T.);
#7911=ORIENTED_EDGE('',*,*,#5685,.T.);
#7912=ORIENTED_EDGE('',*,*,#5729,.T.);
#7913=ORIENTED_EDGE('',*,*,#5660,.F.);
#7914=ORIENTED_EDGE('',*,*,#5743,.F.);
#7915=ORIENTED_EDGE('',*,*,#5743,.T.);
#7916=ORIENTED_EDGE('',*,*,#5744,.T.);
#7917=ORIENTED_EDGE('',*,*,#5745,.T.);
#7918=ORIENTED_EDGE('',*,*,#5744,.F.);
#7919=ORIENTED_EDGE('',*,*,#5745,.F.);
#7920=ORIENTED_EDGE('',*,*,#5746,.F.);
#7921=ORIENTED_EDGE('',*,*,#5746,.T.);
#7922=ORIENTED_EDGE('',*,*,#5747,.T.);
#7923=ORIENTED_EDGE('',*,*,#5748,.F.);
#7924=ORIENTED_EDGE('',*,*,#5749,.F.);
#7925=ORIENTED_EDGE('',*,*,#5747,.F.);
#7926=ORIENTED_EDGE('',*,*,#5750,.F.);
#7927=ORIENTED_EDGE('',*,*,#5751,.F.);
#7928=ORIENTED_EDGE('',*,*,#5716,.F.);
#7929=ORIENTED_EDGE('',*,*,#5697,.T.);
#7930=ORIENTED_EDGE('',*,*,#5752,.T.);
#7931=ORIENTED_EDGE('',*,*,#5719,.T.);
#7932=ORIENTED_EDGE('',*,*,#5703,.F.);
#7933=ORIENTED_EDGE('',*,*,#5753,.F.);
#7934=ORIENTED_EDGE('',*,*,#5754,.F.);
#7935=ORIENTED_EDGE('',*,*,#5755,.F.);
#7936=ORIENTED_EDGE('',*,*,#5721,.T.);
#7937=ORIENTED_EDGE('',*,*,#5752,.F.);
#7938=ORIENTED_EDGE('',*,*,#5756,.F.);
#7939=ORIENTED_EDGE('',*,*,#5755,.T.);
#7940=ORIENTED_EDGE('',*,*,#5734,.T.);
#7941=ORIENTED_EDGE('',*,*,#5667,.T.);
#7942=ORIENTED_EDGE('',*,*,#5730,.T.);
#7943=ORIENTED_EDGE('',*,*,#5695,.T.);
#7944=ORIENTED_EDGE('',*,*,#5757,.T.);
#7945=ORIENTED_EDGE('',*,*,#5758,.T.);
#7946=ORIENTED_EDGE('',*,*,#5759,.T.);
#7947=ORIENTED_EDGE('',*,*,#5760,.T.);
#7948=ORIENTED_EDGE('',*,*,#5761,.T.);
#7949=ORIENTED_EDGE('',*,*,#5762,.T.);
#7950=ORIENTED_EDGE('',*,*,#5763,.T.);
#7951=ORIENTED_EDGE('',*,*,#5764,.T.);
#7952=ORIENTED_EDGE('',*,*,#5750,.T.);
#7953=ORIENTED_EDGE('',*,*,#5756,.T.);
#7954=ORIENTED_EDGE('',*,*,#5754,.T.);
#7955=ORIENTED_EDGE('',*,*,#5765,.T.);
#7956=ORIENTED_EDGE('',*,*,#5766,.T.);
#7957=ORIENTED_EDGE('',*,*,#5767,.T.);
#7958=ORIENTED_EDGE('',*,*,#5768,.T.);
#7959=ORIENTED_EDGE('',*,*,#5769,.T.);
#7960=ORIENTED_EDGE('',*,*,#5753,.T.);
#7961=ORIENTED_EDGE('',*,*,#5706,.T.);
#7962=ORIENTED_EDGE('',*,*,#5724,.F.);
#7963=ORIENTED_EDGE('',*,*,#5708,.F.);
#7964=ORIENTED_EDGE('',*,*,#5770,.T.);
#7965=ORIENTED_EDGE('',*,*,#5765,.F.);
#7966=ORIENTED_EDGE('',*,*,#5654,.T.);
#7967=ORIENTED_EDGE('',*,*,#5741,.T.);
#7968=ORIENTED_EDGE('',*,*,#5651,.F.);
#7969=ORIENTED_EDGE('',*,*,#5739,.T.);
#7970=ORIENTED_EDGE('',*,*,#5740,.T.);
#7971=ORIENTED_EDGE('',*,*,#5671,.T.);
#7972=ORIENTED_EDGE('',*,*,#5737,.T.);
#7973=ORIENTED_EDGE('',*,*,#5649,.F.);
#7974=ORIENTED_EDGE('',*,*,#5771,.F.);
#7975=ORIENTED_EDGE('',*,*,#5771,.T.);
#7976=ORIENTED_EDGE('',*,*,#5772,.T.);
#7977=ORIENTED_EDGE('',*,*,#5773,.T.);
#7978=ORIENTED_EDGE('',*,*,#5772,.F.);
#7979=ORIENTED_EDGE('',*,*,#5773,.F.);
#7980=ORIENTED_EDGE('',*,*,#5774,.F.);
#7981=ORIENTED_EDGE('',*,*,#5774,.T.);
#7982=ORIENTED_EDGE('',*,*,#5775,.T.);
#7983=ORIENTED_EDGE('',*,*,#5776,.F.);
#7984=ORIENTED_EDGE('',*,*,#5777,.F.);
#7985=ORIENTED_EDGE('',*,*,#5778,.F.);
#7986=ORIENTED_EDGE('',*,*,#5779,.F.);
#7987=ORIENTED_EDGE('',*,*,#5775,.F.);
#7988=ORIENTED_EDGE('',*,*,#5767,.F.);
#7989=ORIENTED_EDGE('',*,*,#5780,.T.);
#7990=ORIENTED_EDGE('',*,*,#5742,.T.);
#7991=ORIENTED_EDGE('',*,*,#5656,.T.);
#7992=ORIENTED_EDGE('',*,*,#5738,.T.);
#7993=ORIENTED_EDGE('',*,*,#5681,.T.);
#7994=ORIENTED_EDGE('',*,*,#5768,.F.);
#7995=ORIENTED_EDGE('',*,*,#5780,.F.);
#7996=ORIENTED_EDGE('',*,*,#5766,.F.);
#7997=ORIENTED_EDGE('',*,*,#5770,.F.);
#7998=ORIENTED_EDGE('',*,*,#5707,.F.);
#7999=ORIENTED_EDGE('',*,*,#5711,.F.);
#8000=ORIENTED_EDGE('',*,*,#5726,.F.);
#8001=ORIENTED_EDGE('',*,*,#5700,.F.);
#8002=ORIENTED_EDGE('',*,*,#5713,.F.);
#8003=ORIENTED_EDGE('',*,*,#5781,.F.);
#8004=ORIENTED_EDGE('',*,*,#5751,.T.);
#8005=ORIENTED_EDGE('',*,*,#5769,.F.);
#8006=ORIENTED_EDGE('',*,*,#5781,.T.);
#8007=ORIENTED_EDGE('',*,*,#5715,.T.);
#8008=ORIENTED_EDGE('',*,*,#5722,.F.);
#8009=ORIENTED_EDGE('',*,*,#5717,.F.);
#8010=ORIENTED_EDGE('',*,*,#5761,.F.);
#8011=ORIENTED_EDGE('',*,*,#5782,.T.);
#8012=ORIENTED_EDGE('',*,*,#5783,.F.);
#8013=ORIENTED_EDGE('',*,*,#5782,.F.);
#8014=ORIENTED_EDGE('',*,*,#5762,.F.);
#8015=ORIENTED_EDGE('',*,*,#5784,.T.);
#8016=ORIENTED_EDGE('',*,*,#5785,.F.);
#8017=ORIENTED_EDGE('',*,*,#5784,.F.);
#8018=ORIENTED_EDGE('',*,*,#5763,.F.);
#8019=ORIENTED_EDGE('',*,*,#5786,.T.);
#8020=ORIENTED_EDGE('',*,*,#5787,.F.);
#8021=ORIENTED_EDGE('',*,*,#5786,.F.);
#8022=ORIENTED_EDGE('',*,*,#5764,.F.);
#8023=ORIENTED_EDGE('',*,*,#5788,.T.);
#8024=ORIENTED_EDGE('',*,*,#5789,.F.);
#8025=ORIENTED_EDGE('',*,*,#5788,.F.);
#8026=ORIENTED_EDGE('',*,*,#5725,.F.);
#8027=ORIENTED_EDGE('',*,*,#5790,.T.);
#8028=ORIENTED_EDGE('',*,*,#5776,.T.);
#8029=ORIENTED_EDGE('',*,*,#5779,.T.);
#8030=ORIENTED_EDGE('',*,*,#5791,.T.);
#8031=ORIENTED_EDGE('',*,*,#5792,.F.);
#8032=ORIENTED_EDGE('',*,*,#5791,.F.);
#8033=ORIENTED_EDGE('',*,*,#5778,.T.);
#8034=ORIENTED_EDGE('',*,*,#5777,.T.);
#8035=ORIENTED_EDGE('',*,*,#5790,.F.);
#8036=ORIENTED_EDGE('',*,*,#5748,.T.);
#8037=ORIENTED_EDGE('',*,*,#5749,.T.);
#8038=ORIENTED_EDGE('',*,*,#5793,.T.);
#8039=ORIENTED_EDGE('',*,*,#5794,.T.);
#8040=ORIENTED_EDGE('',*,*,#5760,.F.);
#8041=ORIENTED_EDGE('',*,*,#5795,.F.);
#8042=ORIENTED_EDGE('',*,*,#5796,.T.);
#8043=ORIENTED_EDGE('',*,*,#5795,.T.);
#8044=ORIENTED_EDGE('',*,*,#5759,.F.);
#8045=ORIENTED_EDGE('',*,*,#5797,.F.);
#8046=ORIENTED_EDGE('',*,*,#5798,.T.);
#8047=ORIENTED_EDGE('',*,*,#5797,.T.);
#8048=ORIENTED_EDGE('',*,*,#5758,.F.);
#8049=ORIENTED_EDGE('',*,*,#5799,.F.);
#8050=ORIENTED_EDGE('',*,*,#5800,.T.);
#8051=ORIENTED_EDGE('',*,*,#5799,.T.);
#8052=ORIENTED_EDGE('',*,*,#5757,.F.);
#8053=ORIENTED_EDGE('',*,*,#5794,.F.);
#8054=ORIENTED_EDGE('',*,*,#5800,.F.);
#8055=ORIENTED_EDGE('',*,*,#5793,.F.);
#8056=ORIENTED_EDGE('',*,*,#5796,.F.);
#8057=ORIENTED_EDGE('',*,*,#5798,.F.);
#8058=ORIENTED_EDGE('',*,*,#5792,.T.);
#8059=ORIENTED_EDGE('',*,*,#5789,.T.);
#8060=ORIENTED_EDGE('',*,*,#5787,.T.);
#8061=ORIENTED_EDGE('',*,*,#5785,.T.);
#8062=ORIENTED_EDGE('',*,*,#5783,.T.);
#10304=CYLINDRICAL_SURFACE('',#11637,0.4263);
#10305=CYLINDRICAL_SURFACE('',#11639,0.4263);
#10306=CYLINDRICAL_SURFACE('',#11640,0.4263);
#10307=CYLINDRICAL_SURFACE('',#11642,0.4263);
#10308=CYLINDRICAL_SURFACE('',#11644,0.4263);
#10309=CYLINDRICAL_SURFACE('',#11645,0.4263);
#10310=CYLINDRICAL_SURFACE('',#11647,0.5099);
#10311=CYLINDRICAL_SURFACE('',#11649,0.5099);
#10312=CYLINDRICAL_SURFACE('',#11650,0.5099);
#10313=CYLINDRICAL_SURFACE('',#11651,0.5099);
#10314=CYLINDRICAL_SURFACE('',#11653,0.5099);
#10315=CYLINDRICAL_SURFACE('',#11655,0.5099);
#10316=CYLINDRICAL_SURFACE('',#11656,0.5099);
#10317=CYLINDRICAL_SURFACE('',#11657,0.5099);
#10318=CYLINDRICAL_SURFACE('',#11677,0.5099);
#10319=CYLINDRICAL_SURFACE('',#11678,0.5099);
#10320=CYLINDRICAL_SURFACE('',#11679,0.4263);
#10321=CYLINDRICAL_SURFACE('',#11682,0.4);
#10322=CYLINDRICAL_SURFACE('',#11686,0.2);
#10323=CYLINDRICAL_SURFACE('',#11687,0.7);
#10324=CYLINDRICAL_SURFACE('',#11699,2.4);
#10325=CYLINDRICAL_SURFACE('',#11700,0.4263);
#10326=CYLINDRICAL_SURFACE('',#11703,0.4);
#10327=CYLINDRICAL_SURFACE('',#11707,0.2);
#10328=CYLINDRICAL_SURFACE('',#11710,0.7);
#10329=CYLINDRICAL_SURFACE('',#11711,2.4);
#10330=CYLINDRICAL_SURFACE('',#11712,0.25);
#10331=CYLINDRICAL_SURFACE('',#11714,0.25);
#10332=CYLINDRICAL_SURFACE('',#11716,0.25);
#10333=CYLINDRICAL_SURFACE('',#11718,0.25);
#10334=CYLINDRICAL_SURFACE('',#11720,0.6);
#10769=ADVANCED_FACE('',(#644),#10304,.F.);
#10770=ADVANCED_FACE('',(#645),#10305,.F.);
#10771=ADVANCED_FACE('',(#646),#10306,.F.);
#10772=ADVANCED_FACE('',(#647),#10307,.F.);
#10773=ADVANCED_FACE('',(#648),#10308,.F.);
#10774=ADVANCED_FACE('',(#649),#10309,.F.);
#10775=ADVANCED_FACE('',(#650),#10310,.F.);
#10776=ADVANCED_FACE('',(#651),#10311,.F.);
#10777=ADVANCED_FACE('',(#652),#10312,.F.);
#10778=ADVANCED_FACE('',(#653),#10313,.F.);
#10779=ADVANCED_FACE('',(#654),#10314,.F.);
#10780=ADVANCED_FACE('',(#655),#10315,.F.);
#10781=ADVANCED_FACE('',(#656),#10316,.F.);
#10782=ADVANCED_FACE('',(#657),#10317,.F.);
#10783=ADVANCED_FACE('',(#658),#362,.T.);
#10784=ADVANCED_FACE('',(#659),#363,.T.);
#10785=ADVANCED_FACE('',(#660),#364,.T.);
#10786=ADVANCED_FACE('',(#661),#365,.T.);
#10787=ADVANCED_FACE('',(#662),#366,.T.);
#10788=ADVANCED_FACE('',(#663),#367,.T.);
#10789=ADVANCED_FACE('',(#664),#368,.T.);
#10790=ADVANCED_FACE('',(#665),#369,.T.);
#10791=ADVANCED_FACE('',(#666,#277),#370,.T.);
#10792=ADVANCED_FACE('',(#667),#371,.T.);
#10793=ADVANCED_FACE('',(#668),#10318,.F.);
#10794=ADVANCED_FACE('',(#669),#232,.F.);
#10795=ADVANCED_FACE('',(#670),#233,.F.);
#10796=ADVANCED_FACE('',(#671),#10319,.F.);
#10797=ADVANCED_FACE('',(#672),#234,.F.);
#10798=ADVANCED_FACE('',(#673),#235,.F.);
#10799=ADVANCED_FACE('',(#674),#10320,.F.);
#10800=ADVANCED_FACE('',(#675,#278),#372,.F.);
#10801=ADVANCED_FACE('',(#676),#10321,.F.);
#10802=ADVANCED_FACE('',(#677,#279),#373,.F.);
#10803=ADVANCED_FACE('',(#678),#10322,.F.);
#10804=ADVANCED_FACE('',(#679),#10323,.T.);
#10805=ADVANCED_FACE('',(#680),#374,.F.);
#10806=ADVANCED_FACE('',(#681,#280),#375,.T.);
#10807=ADVANCED_FACE('',(#682,#281,#282,#283,#284,#285),#376,.T.);
#10808=ADVANCED_FACE('',(#683),#10324,.T.);
#10809=ADVANCED_FACE('',(#684),#10325,.F.);
#10810=ADVANCED_FACE('',(#685,#286),#377,.F.);
#10811=ADVANCED_FACE('',(#686),#10326,.F.);
#10812=ADVANCED_FACE('',(#687,#287),#378,.F.);
#10813=ADVANCED_FACE('',(#688),#10327,.F.);
#10814=ADVANCED_FACE('',(#689,#288),#379,.F.);
#10815=ADVANCED_FACE('',(#690),#10328,.T.);
#10816=ADVANCED_FACE('',(#691),#10329,.T.);
#10817=ADVANCED_FACE('',(#692),#10330,.F.);
#10818=ADVANCED_FACE('',(#693),#10331,.F.);
#10819=ADVANCED_FACE('',(#694),#10332,.F.);
#10820=ADVANCED_FACE('',(#695),#10333,.F.);
#10821=ADVANCED_FACE('',(#696,#289),#10334,.F.);
#10822=ADVANCED_FACE('',(#697),#380,.T.);
#10823=ADVANCED_FACE('',(#698),#381,.T.);
#10824=ADVANCED_FACE('',(#699),#382,.T.);
#10825=ADVANCED_FACE('',(#700),#383,.T.);
#10826=ADVANCED_FACE('',(#701,#290,#291,#292,#293,#294),#384,.F.);
#11232=CLOSED_SHELL('',(#10769,#10770,#10771,#10772,#10773,#10774,#10775,
#10776,#10777,#10778,#10779,#10780,#10781,#10782,#10783,#10784,#10785,#10786,
#10787,#10788,#10789,#10790,#10791,#10792,#10793,#10794,#10795,#10796,#10797,
#10798,#10799,#10800,#10801,#10802,#10803,#10804,#10805,#10806,#10807,#10808,
#10809,#10810,#10811,#10812,#10813,#10814,#10815,#10816,#10817,#10818,#10819,
#10820,#10821,#10822,#10823,#10824,#10825,#10826));
#11636=AXIS2_PLACEMENT_3D('',#22260,#12832,#12833);
#11637=AXIS2_PLACEMENT_3D('',#22261,#12834,#12835);
#11638=AXIS2_PLACEMENT_3D('',#22286,#12837,#12838);
#11639=AXIS2_PLACEMENT_3D('',#22318,#12839,#12840);
#11640=AXIS2_PLACEMENT_3D('',#22405,#12842,#12843);
#11641=AXIS2_PLACEMENT_3D('',#22436,#12845,#12846);
#11642=AXIS2_PLACEMENT_3D('',#22474,#12847,#12848);
#11643=AXIS2_PLACEMENT_3D('',#22499,#12850,#12851);
#11644=AXIS2_PLACEMENT_3D('',#22531,#12852,#12853);
#11645=AXIS2_PLACEMENT_3D('',#22618,#12855,#12856);
#11646=AXIS2_PLACEMENT_3D('',#22649,#12858,#12859);
#11647=AXIS2_PLACEMENT_3D('',#22687,#12860,#12861);
#11648=AXIS2_PLACEMENT_3D('',#22697,#12863,#12864);
#11649=AXIS2_PLACEMENT_3D('',#22703,#12865,#12866);
#11650=AXIS2_PLACEMENT_3D('',#22741,#12868,#12869);
#11651=AXIS2_PLACEMENT_3D('',#22777,#12871,#12872);
#11652=AXIS2_PLACEMENT_3D('',#22789,#12874,#12875);
#11653=AXIS2_PLACEMENT_3D('',#22797,#12876,#12877);
#11654=AXIS2_PLACEMENT_3D('',#22807,#12879,#12880);
#11655=AXIS2_PLACEMENT_3D('',#22813,#12881,#12882);
#11656=AXIS2_PLACEMENT_3D('',#22851,#12884,#12885);
#11657=AXIS2_PLACEMENT_3D('',#22887,#12887,#12888);
#11658=AXIS2_PLACEMENT_3D('',#22899,#12890,#12891);
#11659=AXIS2_PLACEMENT_3D('',#22907,#12892,#12893);
#11660=AXIS2_PLACEMENT_3D('',#22910,#12894,#12895);
#11661=AXIS2_PLACEMENT_3D('',#22914,#12898,#12899);
#11662=AXIS2_PLACEMENT_3D('',#22917,#12900,#12901);
#11663=AXIS2_PLACEMENT_3D('',#22921,#12904,#12905);
#11664=AXIS2_PLACEMENT_3D('',#22930,#12910,#12911);
#11665=AXIS2_PLACEMENT_3D('',#22939,#12916,#12917);
#11666=AXIS2_PLACEMENT_3D('',#22941,#12918,#12919);
#11667=AXIS2_PLACEMENT_3D('',#22943,#12921,#12922);
#11668=AXIS2_PLACEMENT_3D('',#22949,#12926,#12927);
#11669=AXIS2_PLACEMENT_3D('',#22955,#12931,#12932);
#11670=AXIS2_PLACEMENT_3D('',#22957,#12933,#12934);
#11671=AXIS2_PLACEMENT_3D('',#22959,#12936,#12937);
#11672=AXIS2_PLACEMENT_3D('',#22961,#12939,#12940);
#11673=AXIS2_PLACEMENT_3D('',#22963,#12942,#12943);
#11674=AXIS2_PLACEMENT_3D('',#22965,#12944,#12945);
#11675=AXIS2_PLACEMENT_3D('',#22966,#12946,#12947);
#11676=AXIS2_PLACEMENT_3D('',#22967,#12948,#12949);
#11677=AXIS2_PLACEMENT_3D('',#22968,#12950,#12951);
#11678=AXIS2_PLACEMENT_3D('',#23761,#12952,#12953);
#11679=AXIS2_PLACEMENT_3D('',#24554,#12954,#12955);
#11680=AXIS2_PLACEMENT_3D('',#24555,#12956,#12957);
#11681=AXIS2_PLACEMENT_3D('',#24557,#12958,#12959);
#11682=AXIS2_PLACEMENT_3D('',#24558,#12960,#12961);
#11683=AXIS2_PLACEMENT_3D('',#24561,#12963,#12964);
#11684=AXIS2_PLACEMENT_3D('',#24562,#12965,#12966);
#11685=AXIS2_PLACEMENT_3D('',#24564,#12967,#12968);
#11686=AXIS2_PLACEMENT_3D('',#24565,#12969,#12970);
#11687=AXIS2_PLACEMENT_3D('',#24605,#12972,#12973);
#11688=AXIS2_PLACEMENT_3D('',#24622,#12975,#12976);
#11689=AXIS2_PLACEMENT_3D('',#24638,#12978,#12979);
#11690=AXIS2_PLACEMENT_3D('',#24639,#12980,#12981);
#11691=AXIS2_PLACEMENT_3D('',#24640,#12982,#12983);
#11692=AXIS2_PLACEMENT_3D('',#24642,#12985,#12986);
#11693=AXIS2_PLACEMENT_3D('',#24652,#12991,#12992);
#11694=AXIS2_PLACEMENT_3D('',#24654,#12993,#12994);
#11695=AXIS2_PLACEMENT_3D('',#24656,#12995,#12996);
#11696=AXIS2_PLACEMENT_3D('',#24658,#12997,#12998);
#11697=AXIS2_PLACEMENT_3D('',#24660,#12999,#13000);
#11698=AXIS2_PLACEMENT_3D('',#24667,#13004,#13005);
#11699=AXIS2_PLACEMENT_3D('',#24668,#13006,#13007);
#11700=AXIS2_PLACEMENT_3D('',#24682,#13008,#13009);
#11701=AXIS2_PLACEMENT_3D('',#24683,#13010,#13011);
#11702=AXIS2_PLACEMENT_3D('',#24685,#13012,#13013);
#11703=AXIS2_PLACEMENT_3D('',#24686,#13014,#13015);
#11704=AXIS2_PLACEMENT_3D('',#24689,#13017,#13018);
#11705=AXIS2_PLACEMENT_3D('',#24690,#13019,#13020);
#11706=AXIS2_PLACEMENT_3D('',#24692,#13021,#13022);
#11707=AXIS2_PLACEMENT_3D('',#24693,#13023,#13024);
#11708=AXIS2_PLACEMENT_3D('',#24739,#13026,#13027);
#11709=AXIS2_PLACEMENT_3D('',#24740,#13028,#13029);
#11710=AXIS2_PLACEMENT_3D('',#24741,#13030,#13031);
#11711=AXIS2_PLACEMENT_3D('',#24754,#13032,#13033);
#11712=AXIS2_PLACEMENT_3D('',#24755,#13034,#13035);
#11713=AXIS2_PLACEMENT_3D('',#24758,#13037,#13038);
#11714=AXIS2_PLACEMENT_3D('',#24759,#13039,#13040);
#11715=AXIS2_PLACEMENT_3D('',#24762,#13042,#13043);
#11716=AXIS2_PLACEMENT_3D('',#24763,#13044,#13045);
#11717=AXIS2_PLACEMENT_3D('',#24766,#13047,#13048);
#11718=AXIS2_PLACEMENT_3D('',#24767,#13049,#13050);
#11719=AXIS2_PLACEMENT_3D('',#24770,#13052,#13053);
#11720=AXIS2_PLACEMENT_3D('',#24771,#13054,#13055);
#11721=AXIS2_PLACEMENT_3D('',#24775,#13058,#13059);
#11722=AXIS2_PLACEMENT_3D('',#24776,#13060,#13061);
#11723=AXIS2_PLACEMENT_3D('',#24782,#13065,#13066);
#11724=AXIS2_PLACEMENT_3D('',#24786,#13069,#13070);
#11725=AXIS2_PLACEMENT_3D('',#24790,#13073,#13074);
#11726=AXIS2_PLACEMENT_3D('',#24792,#13076,#13077);
#12832=DIRECTION('axis',(0.,0.,1.));
#12833=DIRECTION('refdir',(1.,0.,0.));
#12834=DIRECTION('center_axis',(1.,0.,0.));
#12835=DIRECTION('ref_axis',(0.,-0.63690647534225,0.770941075353436));
#12836=DIRECTION('',(1.,0.,0.));
#12837=DIRECTION('center_axis',(-1.,0.,0.));
#12838=DIRECTION('ref_axis',(0.,-1.,0.));
#12839=DIRECTION('center_axis',(1.,0.,0.));
#12840=DIRECTION('ref_axis',(0.,-1.,0.));
#12841=DIRECTION('',(1.,0.,0.));
#12842=DIRECTION('center_axis',(1.,0.,0.));
#12843=DIRECTION('ref_axis',(0.,-0.937046398851017,-0.349204877400562));
#12844=DIRECTION('',(1.,0.,0.));
#12845=DIRECTION('center_axis',(-1.,0.,0.));
#12846=DIRECTION('ref_axis',(0.,-1.,0.));
#12847=DIRECTION('center_axis',(-1.,0.,0.));
#12848=DIRECTION('ref_axis',(0.,0.63690647534225,0.770941075353436));
#12849=DIRECTION('',(-1.,0.,0.));
#12850=DIRECTION('center_axis',(1.,0.,0.));
#12851=DIRECTION('ref_axis',(0.,1.,0.));
#12852=DIRECTION('center_axis',(-1.,0.,0.));
#12853=DIRECTION('ref_axis',(0.,1.,0.));
#12854=DIRECTION('',(-1.,0.,0.));
#12855=DIRECTION('center_axis',(-1.,0.,0.));
#12856=DIRECTION('ref_axis',(0.,0.937046398851017,-0.349204877400562));
#12857=DIRECTION('',(-1.,0.,0.));
#12858=DIRECTION('center_axis',(-1.,0.,0.));
#12859=DIRECTION('ref_axis',(0.,1.,0.));
#12860=DIRECTION('center_axis',(1.,0.,0.));
#12861=DIRECTION('ref_axis',(0.,0.923761774208712,0.382967602429726));
#12862=DIRECTION('',(1.,-1.22464679914735E-16,-1.49975978266186E-32));
#12863=DIRECTION('center_axis',(-1.,0.,0.));
#12864=DIRECTION('ref_axis',(0.,-1.,0.));
#12865=DIRECTION('center_axis',(1.,0.,0.));
#12866=DIRECTION('ref_axis',(0.,-1.,0.));
#12867=DIRECTION('',(1.,-1.22464679914735E-16,-1.49975978266186E-32));
#12868=DIRECTION('center_axis',(1.,0.,0.));
#12869=DIRECTION('ref_axis',(0.,-1.,0.));
#12870=DIRECTION('',(1.,-1.22464679914735E-16,-1.49975978266186E-32));
#12871=DIRECTION('center_axis',(1.,0.,0.));
#12872=DIRECTION('ref_axis',(0.,0.608513123927572,-0.79354380975968));
#12873=DIRECTION('',(1.,-1.22464679914735E-16,-1.49975978266186E-32));
#12874=DIRECTION('center_axis',(1.,0.,0.));
#12875=DIRECTION('ref_axis',(0.,-1.,0.));
#12876=DIRECTION('center_axis',(-1.,0.,0.));
#12877=DIRECTION('ref_axis',(0.,-0.923761774208712,0.382967602429726));
#12878=DIRECTION('',(-1.,1.22464679914735E-16,-1.49975978266186E-32));
#12879=DIRECTION('center_axis',(1.,0.,0.));
#12880=DIRECTION('ref_axis',(0.,1.,0.));
#12881=DIRECTION('center_axis',(-1.,0.,0.));
#12882=DIRECTION('ref_axis',(0.,1.,0.));
#12883=DIRECTION('',(-1.,1.22464679914735E-16,-1.49975978266186E-32));
#12884=DIRECTION('center_axis',(-1.,0.,0.));
#12885=DIRECTION('ref_axis',(0.,1.,0.));
#12886=DIRECTION('',(-1.,1.22464679914735E-16,-1.49975978266186E-32));
#12887=DIRECTION('center_axis',(-1.,0.,0.));
#12888=DIRECTION('ref_axis',(0.,-0.608513123927572,-0.79354380975968));
#12889=DIRECTION('',(-1.,1.22464679914735E-16,-1.49975978266186E-32));
#12890=DIRECTION('center_axis',(-1.,0.,0.));
#12891=DIRECTION('ref_axis',(0.,1.,0.));
#12892=DIRECTION('center_axis',(1.,0.,0.));
#12893=DIRECTION('ref_axis',(0.,1.,0.));
#12894=DIRECTION('center_axis',(1.,0.,0.));
#12895=DIRECTION('ref_axis',(0.,0.,-1.));
#12896=DIRECTION('',(0.,0.,1.));
#12897=DIRECTION('',(0.,1.,0.));
#12898=DIRECTION('center_axis',(-1.,0.,0.));
#12899=DIRECTION('ref_axis',(0.,-1.,0.));
#12900=DIRECTION('center_axis',(1.,0.,0.));
#12901=DIRECTION('ref_axis',(0.,0.,-1.));
#12902=DIRECTION('',(0.,-1.,0.));
#12903=DIRECTION('',(0.,0.,1.));
#12904=DIRECTION('center_axis',(-1.6809537598482E-15,1.,0.));
#12905=DIRECTION('ref_axis',(-1.,-1.6809537598482E-15,0.));
#12906=DIRECTION('',(-1.,0.,0.));
#12907=DIRECTION('',(0.,0.,1.));
#12908=DIRECTION('',(-1.,-1.6809537598482E-15,0.));
#12909=DIRECTION('',(0.,0.,1.));
#12910=DIRECTION('center_axis',(3.3619075196964E-16,1.,0.));
#12911=DIRECTION('ref_axis',(-1.,3.3619075196964E-16,0.));
#12912=DIRECTION('',(-1.,0.,0.));
#12913=DIRECTION('',(0.,0.,1.));
#12914=DIRECTION('',(-1.,3.3619075196964E-16,0.));
#12915=DIRECTION('',(0.,0.,1.));
#12916=DIRECTION('center_axis',(-1.,0.,0.));
#12917=DIRECTION('ref_axis',(0.,-1.,0.));
#12918=DIRECTION('center_axis',(1.,0.,0.));
#12919=DIRECTION('ref_axis',(0.,0.,-1.));
#12920=DIRECTION('',(0.,-1.,0.));
#12921=DIRECTION('center_axis',(2.35333526378748E-15,-1.,0.));
#12922=DIRECTION('ref_axis',(1.,2.35333526378748E-15,0.));
#12923=DIRECTION('',(1.,0.,0.));
#12924=DIRECTION('',(1.,2.35333526378748E-15,0.));
#12925=DIRECTION('',(0.,0.,1.));
#12926=DIRECTION('center_axis',(-3.3619075196964E-16,-1.,0.));
#12927=DIRECTION('ref_axis',(1.,-3.3619075196964E-16,0.));
#12928=DIRECTION('',(1.,0.,0.));
#12929=DIRECTION('',(0.,0.,1.));
#12930=DIRECTION('',(1.,-3.3619075196964E-16,0.));
#12931=DIRECTION('center_axis',(1.,0.,0.));
#12932=DIRECTION('ref_axis',(0.,1.,0.));
#12933=DIRECTION('center_axis',(1.,0.,0.));
#12934=DIRECTION('ref_axis',(0.,0.,-1.));
#12935=DIRECTION('',(0.,1.,0.));
#12936=DIRECTION('center_axis',(0.,0.,1.));
#12937=DIRECTION('ref_axis',(-1.,0.,0.));
#12938=DIRECTION('',(0.,-1.,0.));
#12939=DIRECTION('center_axis',(0.,0.,1.));
#12940=DIRECTION('ref_axis',(0.970931683144254,0.239356776939084,0.));
#12941=DIRECTION('',(0.,1.,0.));
#12942=DIRECTION('center_axis',(0.,0.,1.));
#12943=DIRECTION('ref_axis',(-0.970931683144254,-0.239356776939084,0.));
#12944=DIRECTION('center_axis',(0.,0.,-1.));
#12945=DIRECTION('ref_axis',(-1.,0.,0.));
#12946=DIRECTION('center_axis',(1.,0.,0.));
#12947=DIRECTION('ref_axis',(0.,0.,-1.));
#12948=DIRECTION('center_axis',(1.,0.,0.));
#12949=DIRECTION('ref_axis',(0.,0.,-1.));
#12950=DIRECTION('center_axis',(-1.,0.,0.));
#12951=DIRECTION('ref_axis',(0.,1.,0.));
#12952=DIRECTION('center_axis',(1.,0.,0.));
#12953=DIRECTION('ref_axis',(0.,-1.,0.));
#12954=DIRECTION('center_axis',(-1.,0.,0.));
#12955=DIRECTION('ref_axis',(0.,1.,0.));
#12956=DIRECTION('center_axis',(-1.,0.,0.));
#12957=DIRECTION('ref_axis',(0.,1.,0.));
#12958=DIRECTION('center_axis',(1.,0.,0.));
#12959=DIRECTION('ref_axis',(0.,1.,0.));
#12960=DIRECTION('center_axis',(-1.,0.,0.));
#12961=DIRECTION('ref_axis',(0.,1.,0.));
#12962=DIRECTION('',(-1.,0.,0.));
#12963=DIRECTION('center_axis',(-1.,0.,0.));
#12964=DIRECTION('ref_axis',(0.,1.,0.));
#12965=DIRECTION('center_axis',(-1.,0.,0.));
#12966=DIRECTION('ref_axis',(0.,1.,0.));
#12967=DIRECTION('center_axis',(1.,0.,0.));
#12968=DIRECTION('ref_axis',(0.,1.,0.));
#12969=DIRECTION('center_axis',(-1.,0.,0.));
#12970=DIRECTION('ref_axis',(0.,1.,0.));
#12971=DIRECTION('',(-1.,0.,0.));
#12972=DIRECTION('center_axis',(1.,0.,0.));
#12973=DIRECTION('ref_axis',(0.,1.22464679914735E-16,1.));
#12974=DIRECTION('',(1.,0.,0.));
#12975=DIRECTION('center_axis',(1.,0.,0.));
#12976=DIRECTION('ref_axis',(0.,0.,-1.));
#12977=DIRECTION('',(-1.,0.,0.));
#12978=DIRECTION('center_axis',(1.,0.,0.));
#12979=DIRECTION('ref_axis',(0.,0.,-1.));
#12980=DIRECTION('center_axis',(1.,0.,0.));
#12981=DIRECTION('ref_axis',(0.,0.,-1.));
#12982=DIRECTION('center_axis',(1.,0.,0.));
#12983=DIRECTION('ref_axis',(0.,0.,-1.));
#12984=DIRECTION('',(0.,-1.,0.));
#12985=DIRECTION('center_axis',(0.,0.,1.));
#12986=DIRECTION('ref_axis',(1.,0.,0.));
#12987=DIRECTION('',(0.,-1.,0.));
#12988=DIRECTION('',(1.,0.,0.));
#12989=DIRECTION('',(0.,1.,0.));
#12990=DIRECTION('',(-1.,0.,0.));
#12991=DIRECTION('center_axis',(0.,0.,-1.));
#12992=DIRECTION('ref_axis',(1.,0.,0.));
#12993=DIRECTION('center_axis',(0.,0.,-1.));
#12994=DIRECTION('ref_axis',(1.,0.,0.));
#12995=DIRECTION('center_axis',(0.,0.,-1.));
#12996=DIRECTION('ref_axis',(1.,0.,0.));
#12997=DIRECTION('center_axis',(0.,0.,-1.));
#12998=DIRECTION('ref_axis',(1.,0.,0.));
#12999=DIRECTION('center_axis',(0.,0.,-1.));
#13000=DIRECTION('ref_axis',(1.,0.,0.));
#13001=DIRECTION('',(-1.,0.,0.));
#13002=DIRECTION('',(0.,1.,0.));
#13003=DIRECTION('',(1.,0.,0.));
#13004=DIRECTION('center_axis',(0.,0.,-1.));
#13005=DIRECTION('ref_axis',(1.,0.,0.));
#13006=DIRECTION('center_axis',(0.,0.,1.));
#13007=DIRECTION('ref_axis',(1.,0.,0.));
#13008=DIRECTION('center_axis',(1.,0.,0.));
#13009=DIRECTION('ref_axis',(0.,-1.,0.));
#13010=DIRECTION('center_axis',(1.,0.,0.));
#13011=DIRECTION('ref_axis',(0.,-1.,0.));
#13012=DIRECTION('center_axis',(-1.,0.,0.));
#13013=DIRECTION('ref_axis',(0.,-1.,0.));
#13014=DIRECTION('center_axis',(1.,0.,0.));
#13015=DIRECTION('ref_axis',(0.,-1.,0.));
#13016=DIRECTION('',(1.,0.,0.));
#13017=DIRECTION('center_axis',(1.,0.,0.));
#13018=DIRECTION('ref_axis',(0.,-1.,0.));
#13019=DIRECTION('center_axis',(1.,0.,0.));
#13020=DIRECTION('ref_axis',(0.,-1.,0.));
#13021=DIRECTION('center_axis',(-1.,0.,0.));
#13022=DIRECTION('ref_axis',(0.,-1.,0.));
#13023=DIRECTION('center_axis',(1.,0.,0.));
#13024=DIRECTION('ref_axis',(0.,-1.,0.));
#13025=DIRECTION('',(1.,0.,0.));
#13026=DIRECTION('center_axis',(1.,0.,0.));
#13027=DIRECTION('ref_axis',(0.,0.,-1.));
#13028=DIRECTION('center_axis',(-1.,0.,0.));
#13029=DIRECTION('ref_axis',(0.,0.,-1.));
#13030=DIRECTION('center_axis',(-1.,0.,0.));
#13031=DIRECTION('ref_axis',(0.,1.22464679914735E-16,1.));
#13032=DIRECTION('center_axis',(0.,0.,1.));
#13033=DIRECTION('ref_axis',(1.,0.,0.));
#13034=DIRECTION('center_axis',(0.,0.,-1.));
#13035=DIRECTION('ref_axis',(1.,0.,0.));
#13036=DIRECTION('',(0.,0.,-1.));
#13037=DIRECTION('center_axis',(0.,0.,1.));
#13038=DIRECTION('ref_axis',(1.,0.,0.));
#13039=DIRECTION('center_axis',(0.,0.,-1.));
#13040=DIRECTION('ref_axis',(1.,0.,0.));
#13041=DIRECTION('',(0.,0.,-1.));
#13042=DIRECTION('center_axis',(0.,0.,1.));
#13043=DIRECTION('ref_axis',(1.,0.,0.));
#13044=DIRECTION('center_axis',(0.,0.,-1.));
#13045=DIRECTION('ref_axis',(1.,0.,0.));
#13046=DIRECTION('',(0.,0.,-1.));
#13047=DIRECTION('center_axis',(0.,0.,1.));
#13048=DIRECTION('ref_axis',(1.,0.,0.));
#13049=DIRECTION('center_axis',(0.,0.,-1.));
#13050=DIRECTION('ref_axis',(1.,0.,0.));
#13051=DIRECTION('',(0.,0.,-1.));
#13052=DIRECTION('center_axis',(0.,0.,1.));
#13053=DIRECTION('ref_axis',(1.,0.,0.));
#13054=DIRECTION('center_axis',(0.,0.,-1.));
#13055=DIRECTION('ref_axis',(1.,0.,0.));
#13056=DIRECTION('',(0.,0.,-1.));
#13057=DIRECTION('',(0.,0.,-1.));
#13058=DIRECTION('center_axis',(0.,0.,1.));
#13059=DIRECTION('ref_axis',(1.,0.,0.));
#13060=DIRECTION('center_axis',(0.,1.,0.));
#13061=DIRECTION('ref_axis',(-1.,0.,0.));
#13062=DIRECTION('',(-1.,0.,0.));
#13063=DIRECTION('',(0.,0.,1.));
#13064=DIRECTION('',(0.,0.,1.));
#13065=DIRECTION('center_axis',(1.,0.,0.));
#13066=DIRECTION('ref_axis',(0.,1.,0.));
#13067=DIRECTION('',(0.,1.,0.));
#13068=DIRECTION('',(0.,0.,1.));
#13069=DIRECTION('center_axis',(0.,-1.,0.));
#13070=DIRECTION('ref_axis',(1.,0.,0.));
#13071=DIRECTION('',(1.,0.,0.));
#13072=DIRECTION('',(0.,0.,1.));
#13073=DIRECTION('center_axis',(-1.,0.,0.));
#13074=DIRECTION('ref_axis',(0.,-1.,0.));
#13075=DIRECTION('',(0.,-1.,0.));
#13076=DIRECTION('center_axis',(0.,0.,1.));
#13077=DIRECTION('ref_axis',(1.,0.,0.));
#22260=CARTESIAN_POINT('',(0.,0.,0.));
#22261=CARTESIAN_POINT('Origin',(-2.35,0.,6.4));
#22262=CARTESIAN_POINT('',(-2.2079681670589,0.426326761040182,6.40000738455106));
#22263=CARTESIAN_POINT('',(-2.16703183294109,0.426272942583651,6.39999240784429));
#22264=CARTESIAN_POINT('',(-2.35,0.4263,6.4));
#22265=CARTESIAN_POINT('',(-2.1,-0.402774227945242,6.53965891057542));
#22266=CARTESIAN_POINT('Ctrl Pts',(-2.16703183294109,0.426272942583651,
6.39999240784429));
#22267=CARTESIAN_POINT('Ctrl Pts',(-2.16455261625436,0.426244983352413,
6.44427071500844));
#22268=CARTESIAN_POINT('Ctrl Pts',(-2.16207339956763,0.419380394763561,
6.488557477259));
#22269=CARTESIAN_POINT('Ctrl Pts',(-2.1595941828809,0.405813684403497,6.53068600993882));
#22270=CARTESIAN_POINT('Ctrl Pts',(-2.1556212373555,0.384073026756357,6.59819699689588));
#22271=CARTESIAN_POINT('Ctrl Pts',(-2.15164829183011,0.34512127171195,6.66016563463643));
#22272=CARTESIAN_POINT('Ctrl Pts',(-2.14767534630472,0.293711532789595,
6.70902687081076));
#22273=CARTESIAN_POINT('Ctrl Pts',(-2.14370240077932,0.242301793867241,
6.75788810698509));
#22274=CARTESIAN_POINT('Ctrl Pts',(-2.13972945525393,0.178434071066939,
6.7936419415932));
#22275=CARTESIAN_POINT('Ctrl Pts',(-2.13575650972854,0.10990720362842,6.81192661575963));
#22276=CARTESIAN_POINT('Ctrl Pts',(-2.13178356420314,0.0413803361899007,
6.83021128992606));
#22277=CARTESIAN_POINT('Ctrl Pts',(-2.12781061867775,-0.031805675886835,
6.83102680365082));
#22278=CARTESIAN_POINT('Ctrl Pts',(-2.12383767315236,-0.100723579247557,
6.81426824831305));
#22279=CARTESIAN_POINT('Ctrl Pts',(-2.11986472762697,-0.169641482608279,
6.79750969297527));
#22280=CARTESIAN_POINT('Ctrl Pts',(-2.11589178210157,-0.234291277252986,
6.76317706857497));
#22281=CARTESIAN_POINT('Ctrl Pts',(-2.11191883657618,-0.286764012116973,
6.71547162888731));
#22282=CARTESIAN_POINT('Ctrl Pts',(-2.10794589105079,-0.33923674698096,
6.66776618919964));
#22283=CARTESIAN_POINT('Ctrl Pts',(-2.10397294552539,-0.379532422064226,
6.60668793422461));
#22284=CARTESIAN_POINT('Ctrl Pts',(-2.1,-0.402774227945242,6.53965891057542));
#22285=CARTESIAN_POINT('',(-2.1,-0.0804421690761202,5.98132232055468));
#22286=CARTESIAN_POINT('Origin',(-2.1,0.,6.4));
#22287=CARTESIAN_POINT('Ctrl Pts',(-2.1,-0.0804421690761202,5.98132232055468));
#22288=CARTESIAN_POINT('Ctrl Pts',(-2.10377590012555,-0.14663424989577,
5.99407142716487));
#22289=CARTESIAN_POINT('Ctrl Pts',(-2.1075518002511,-0.209775930044154,
6.02277117104005));
#22290=CARTESIAN_POINT('Ctrl Pts',(-2.11132770037664,-0.262848123123102,
6.06432984686491));
#22291=CARTESIAN_POINT('Ctrl Pts',(-2.11530064590204,-0.318689889325856,
6.10805726275774));
#22292=CARTESIAN_POINT('Ctrl Pts',(-2.11927359142743,-0.363383793828482,
6.16602071609696));
#22293=CARTESIAN_POINT('Ctrl Pts',(-2.12324653695282,-0.391474229567156,
6.2311459484684));
#22294=CARTESIAN_POINT('Ctrl Pts',(-2.12721948247822,-0.41956466530583,
6.29627118083984));
#22295=CARTESIAN_POINT('Ctrl Pts',(-2.13119242800361,-0.431051632280552,
6.36855819224351));
#22296=CARTESIAN_POINT('Ctrl Pts',(-2.135165373529,-0.4245331350138,6.43918322464256));
#22297=CARTESIAN_POINT('Ctrl Pts',(-2.1391383190544,-0.418014637747048,
6.50980825704162));
#22298=CARTESIAN_POINT('Ctrl Pts',(-2.14311126457979,-0.393490676238824,
6.57877131043605));
#22299=CARTESIAN_POINT('Ctrl Pts',(-2.14708421010518,-0.353954606539213,
6.63765488796442));
#22300=CARTESIAN_POINT('Ctrl Pts',(-2.15105715563058,-0.314418536839601,
6.69653846549279));
#22301=CARTESIAN_POINT('Ctrl Pts',(-2.15503010115597,-0.259870358948601,
6.74534256715509));
#22302=CARTESIAN_POINT('Ctrl Pts',(-2.15900304668136,-0.196968276722384,
6.77811005889651));
#22303=CARTESIAN_POINT('Ctrl Pts',(-2.16297599220675,-0.134066194496165,
6.81087755063794));
#22304=CARTESIAN_POINT('Ctrl Pts',(-2.16694893773215,-0.0628102079347276,
6.8276084324585));
#22305=CARTESIAN_POINT('Ctrl Pts',(-2.17092188325754,0.00810215006175566,
6.82626056070251));
#22306=CARTESIAN_POINT('Ctrl Pts',(-2.17489482878293,0.0790145080582389,
6.82491268894653));
#22307=CARTESIAN_POINT('Ctrl Pts',(-2.17886777430833,0.149583237489768,
6.805486063614));
#22308=CARTESIAN_POINT('Ctrl Pts',(-2.18284071983372,0.211194676111135,
6.77035189196174));
#22309=CARTESIAN_POINT('Ctrl Pts',(-2.18681366535911,0.272806114732501,
6.73521772030948));
#22310=CARTESIAN_POINT('Ctrl Pts',(-2.19078661088451,0.325460262543706,
6.68437600233748));
#22311=CARTESIAN_POINT('Ctrl Pts',(-2.1947595564099,0.362730128342859,6.62403251342481));
#22312=CARTESIAN_POINT('Ctrl Pts',(-2.19873250193529,0.399999994142011,
6.56368902451214));
#22313=CARTESIAN_POINT('Ctrl Pts',(-2.20270544746069,0.421885577929111,
6.4938437646588));
#22314=CARTESIAN_POINT('Ctrl Pts',(-2.20667839298608,0.425715512458415,
6.42302208016789));
#22315=CARTESIAN_POINT('Ctrl Pts',(-2.20710831767702,0.426129961488313,
6.41535824722023));
#22316=CARTESIAN_POINT('Ctrl Pts',(-2.20753824236796,0.426332977570519,
6.40768298027005));
#22317=CARTESIAN_POINT('Ctrl Pts',(-2.2079681670589,0.426326761040182,6.40000738455106));
#22318=CARTESIAN_POINT('Origin',(-2.35,0.,6.4));
#22319=CARTESIAN_POINT('',(-2.3579681670589,0.426284649716722,6.39998978457651));
#22320=CARTESIAN_POINT('',(-2.31703183294109,0.426305653513777,6.40001091236462));
#22321=CARTESIAN_POINT('',(-2.35,0.4263,6.4));
#22322=CARTESIAN_POINT('Ctrl Pts',(-2.31703183294109,0.426305653513777,
6.40001091236462));
#22323=CARTESIAN_POINT('Ctrl Pts',(-2.31620090808447,0.426321019141741,
6.41484782419694));
#22324=CARTESIAN_POINT('Ctrl Pts',(-2.31536998322785,0.425561575912188,
6.42968317075982));
#22325=CARTESIAN_POINT('Ctrl Pts',(-2.31453905837123,0.42401549701117,6.44443607928542));
#22326=CARTESIAN_POINT('Ctrl Pts',(-2.31056611284584,0.416623147146128,
6.51497495105736));
#22327=CARTESIAN_POINT('Ctrl Pts',(-2.30659316732044,0.391247250234886,
6.58362917867256));
#22328=CARTESIAN_POINT('Ctrl Pts',(-2.30262022179505,0.350985201969758,
6.6420187902307));
#22329=CARTESIAN_POINT('Ctrl Pts',(-2.29864727626966,0.310723153704629,
6.70040840178883));
#22330=CARTESIAN_POINT('Ctrl Pts',(-2.29467433074426,0.255574954085614,
6.74853339728991));
#22331=CARTESIAN_POINT('Ctrl Pts',(-2.29070138521887,0.192272021883084,
6.78051961378245));
#22332=CARTESIAN_POINT('Ctrl Pts',(-2.28672843969348,0.128969089680553,
6.81250583027498));
#22333=CARTESIAN_POINT('Ctrl Pts',(-2.28275549416808,0.0575114248945075,
6.82835326775898));
#22334=CARTESIAN_POINT('Ctrl Pts',(-2.27878254864269,-0.013378811171034,
6.82612757973448));
#22335=CARTESIAN_POINT('Ctrl Pts',(-2.2748096031173,-0.0842690472365756,
6.82390189170998));
#22336=CARTESIAN_POINT('Ctrl Pts',(-2.27083665759191,-0.154591854581613,
6.80360307817698));
#22337=CARTESIAN_POINT('Ctrl Pts',(-2.26686371206651,-0.215763594163553,
6.76770882270937));
#22338=CARTESIAN_POINT('Ctrl Pts',(-2.26289076654112,-0.276935333745493,
6.73181456724177));
#22339=CARTESIAN_POINT('Ctrl Pts',(-2.25891782101573,-0.328956005564335,
6.68032486983957));
#22340=CARTESIAN_POINT('Ctrl Pts',(-2.25494487549033,-0.365475937036552,
6.61952459179481));
#22341=CARTESIAN_POINT('Ctrl Pts',(-2.25097192996494,-0.401995868508769,
6.55872431375006));
#22342=CARTESIAN_POINT('Ctrl Pts',(-2.24699898443955,-0.423015059634361,
6.48861345506275));
#22343=CARTESIAN_POINT('Ctrl Pts',(-2.24302603891415,-0.425967899647639,
6.4177497824262));
#22344=CARTESIAN_POINT('Ctrl Pts',(-2.23905309338876,-0.428920739660916,
6.34688610978966));
#22345=CARTESIAN_POINT('Ctrl Pts',(-2.23508014786337,-0.413807228561879,
6.27526962320388));
#22346=CARTESIAN_POINT('Ctrl Pts',(-2.23110720233797,-0.382472123166929,
6.21164187477894));
#22347=CARTESIAN_POINT('Ctrl Pts',(-2.22713425681258,-0.35113701777198,
6.14801412635401));
#22348=CARTESIAN_POINT('Ctrl Pts',(-2.22316131128719,-0.303580318081118,
6.09237511608992));
#22349=CARTESIAN_POINT('Ctrl Pts',(-2.2191883657618,-0.245606834378852,
6.05151616024381));
#22350=CARTESIAN_POINT('Ctrl Pts',(-2.2152154202364,-0.187633350676587,
6.0106572043977));
#22351=CARTESIAN_POINT('Ctrl Pts',(-2.21124247471101,-0.119243082962917,
5.98457830296956));
#22352=CARTESIAN_POINT('Ctrl Pts',(-2.20726952918561,-0.0487837540878456,
5.97646268493538));
#22353=CARTESIAN_POINT('Ctrl Pts',(-2.20329658366022,0.0216755747872263,
5.96834706690119));
#22354=CARTESIAN_POINT('Ctrl Pts',(-2.19932363813483,0.0942039648236993,
5.97819473226094));
#22355=CARTESIAN_POINT('Ctrl Pts',(-2.19535069260944,0.159948497199684,
6.00480361749332));
#22356=CARTESIAN_POINT('Ctrl Pts',(-2.19137774708404,0.225693029575669,
6.03141250272569));
#22357=CARTESIAN_POINT('Ctrl Pts',(-2.18740480155865,0.284653704291167,
6.07478260783069));
#22358=CARTESIAN_POINT('Ctrl Pts',(-2.18343185603326,0.329633888906202,
6.12962026666635));
#22359=CARTESIAN_POINT('Ctrl Pts',(-2.17945891050786,0.374614073521237,
6.184457925502));
#22360=CARTESIAN_POINT('Ctrl Pts',(-2.17548596498247,0.40561376803581,6.25076313806833));
#22361=CARTESIAN_POINT('Ctrl Pts',(-2.17151301945708,0.41884883516816,6.32044241243827));
#22362=CARTESIAN_POINT('Ctrl Pts',(-2.17001929061842,0.423824891681104,
6.34664008892744));
#22363=CARTESIAN_POINT('Ctrl Pts',(-2.16852556177975,0.426289788029324,
6.37331471375964));
#22364=CARTESIAN_POINT('Ctrl Pts',(-2.16703183294109,0.426272942583651,
6.39999240784429));
#22365=CARTESIAN_POINT('Ctrl Pts',(-2.2079681670589,0.426326761040182,6.40000738455106));
#22366=CARTESIAN_POINT('Ctrl Pts',(-2.21151118789336,0.426275530448026,
6.3367525956958));
#22367=CARTESIAN_POINT('Ctrl Pts',(-2.21505420872781,0.412014367364063,
6.27347547866508));
#22368=CARTESIAN_POINT('Ctrl Pts',(-2.21859722956226,0.384774767183445,
6.21639147031607));
#22369=CARTESIAN_POINT('Ctrl Pts',(-2.22257017508765,0.354229802107662,
6.15238065408364));
#22370=CARTESIAN_POINT('Ctrl Pts',(-2.22654312061304,0.307365586684588,
6.09615713074728));
#22371=CARTESIAN_POINT('Ctrl Pts',(-2.23051606613844,0.249902392017012,
6.05458357301381));
#22372=CARTESIAN_POINT('Ctrl Pts',(-2.23448901166383,0.192439197349434,
6.01301001528034));
#22373=CARTESIAN_POINT('Ctrl Pts',(-2.23846195718922,0.124377023437354,
5.98608642314976));
#22374=CARTESIAN_POINT('Ctrl Pts',(-2.24243490271462,0.0540235759521597,
5.97709910512957));
#22375=CARTESIAN_POINT('Ctrl Pts',(-2.24640784824001,-0.0163298715330345,
5.96811178710938));
#22376=CARTESIAN_POINT('Ctrl Pts',(-2.2503807937654,-0.0889745925913431,
5.97706074319959));
#22377=CARTESIAN_POINT('Ctrl Pts',(-2.2543537392908,-0.155043533545503,
6.00285365883444));
#22378=CARTESIAN_POINT('Ctrl Pts',(-2.25832668481619,-0.221112474499663,
6.02864657446929));
#22379=CARTESIAN_POINT('Ctrl Pts',(-2.26229963034158,-0.280605635349674,
6.07128344964878));
#22380=CARTESIAN_POINT('Ctrl Pts',(-2.26627257586698,-0.326261248855651,
6.1255600045331));
#22381=CARTESIAN_POINT('Ctrl Pts',(-2.27024552139237,-0.371916862361629,
6.17983655941743));
#22382=CARTESIAN_POINT('Ctrl Pts',(-2.27421846691776,-0.403734928523572,
6.24575279400659));
#22383=CARTESIAN_POINT('Ctrl Pts',(-2.27819141244315,-0.417831717081485,
6.31526293721211));
#22384=CARTESIAN_POINT('Ctrl Pts',(-2.28216435796855,-0.431928505639397,
6.38477308041763));
#22385=CARTESIAN_POINT('Ctrl Pts',(-2.28613730349394,-0.42830401659328,
6.45787713223949));
#22386=CARTESIAN_POINT('Ctrl Pts',(-2.29011024901934,-0.407400657020557,
6.52565197280568));
#22387=CARTESIAN_POINT('Ctrl Pts',(-2.29408319454473,-0.386497297447833,
6.59342681337187));
#22388=CARTESIAN_POINT('Ctrl Pts',(-2.29805614007012,-0.348315067348504,
6.65587244268238));
#22389=CARTESIAN_POINT('Ctrl Pts',(-2.30202908559551,-0.297514510269819,
6.70536671362482));
#22390=CARTESIAN_POINT('Ctrl Pts',(-2.30600203112091,-0.246713953191133,
6.75486098456727));
#22391=CARTESIAN_POINT('Ctrl Pts',(-2.3099749766463,-0.18329506913309,6.79140389714166));
#22392=CARTESIAN_POINT('Ctrl Pts',(-2.31394792217169,-0.114998801196742,
6.81053500378618));
#22393=CARTESIAN_POINT('Ctrl Pts',(-2.31792086769709,-0.0467025332603938,
6.8296661104307));
#22394=CARTESIAN_POINT('Ctrl Pts',(-2.32189381322248,0.0264711185542592,
6.83138541114536));
#22395=CARTESIAN_POINT('Ctrl Pts',(-2.32586675874787,0.0955905389447022,
6.81548304715754));
#22396=CARTESIAN_POINT('Ctrl Pts',(-2.32983970427327,0.164709959335145,
6.79958068316972));
#22397=CARTESIAN_POINT('Ctrl Pts',(-2.33381264979866,0.229775148301378,
6.76605665447942));
#22398=CARTESIAN_POINT('Ctrl Pts',(-2.33778559532405,0.282844213879021,
6.71900292206431));
#22399=CARTESIAN_POINT('Ctrl Pts',(-2.34175854084945,0.335913279456664,
6.67194918964919));
#22400=CARTESIAN_POINT('Ctrl Pts',(-2.34573148637484,0.376986221645717,
6.61136575350926));
#22401=CARTESIAN_POINT('Ctrl Pts',(-2.34970443190023,0.40104965502802,6.54464746044443));
#22402=CARTESIAN_POINT('Ctrl Pts',(-2.35245901028646,0.417733652598481,
6.49838939653));
#22403=CARTESIAN_POINT('Ctrl Pts',(-2.35521358867268,0.42624097353767,6.44918223268425));
#22404=CARTESIAN_POINT('Ctrl Pts',(-2.3579681670589,0.426284649716722,6.39998978457651));
#22405=CARTESIAN_POINT('Origin',(-2.35,0.,6.4));
#22406=CARTESIAN_POINT('',(-2.50796816705891,0.426290360635438,6.40001083203199));
#22407=CARTESIAN_POINT('',(-2.46703183294109,0.426306423912841,6.39998913682467));
#22408=CARTESIAN_POINT('',(-2.35,0.4263,6.4));
#22409=CARTESIAN_POINT('',(-2.6,-0.32233527839578,6.67898325810255));
#22410=CARTESIAN_POINT('Ctrl Pts',(-2.50796816705891,0.426290360635438,
6.40001083203199));
#22411=CARTESIAN_POINT('Ctrl Pts',(-2.51083482602818,0.426241188929821,
6.34881879719149));
#22412=CARTESIAN_POINT('Ctrl Pts',(-2.51370148499746,0.417011809736389,
6.29760951317986));
#22413=CARTESIAN_POINT('Ctrl Pts',(-2.51656814396674,0.398972669717071,
6.24971854193924));
#22414=CARTESIAN_POINT('Ctrl Pts',(-2.52054108949214,0.373971955858283,
6.18334572887142));
#22415=CARTESIAN_POINT('Ctrl Pts',(-2.52451403501753,0.332049803576913,
6.12334659907732));
#22416=CARTESIAN_POINT('Ctrl Pts',(-2.52848698054292,0.278323314671085,
6.07704505632467));
#22417=CARTESIAN_POINT('Ctrl Pts',(-2.53245992606832,0.224596825765257,
6.03074351357203));
#22418=CARTESIAN_POINT('Ctrl Pts',(-2.53643287159371,0.159066000234972,
5.99813955786084));
#22419=CARTESIAN_POINT('Ctrl Pts',(-2.5404058171191,0.089729440237079,5.98321202621739));
#22420=CARTESIAN_POINT('Ctrl Pts',(-2.5443787626445,0.0203928802391868,
5.96828449457393));
#22421=CARTESIAN_POINT('Ctrl Pts',(-2.54835170816989,-0.0527494142263132,
5.97103338699821));
#22422=CARTESIAN_POINT('Ctrl Pts',(-2.55232465369528,-0.120769354923407,
5.99112490728642));
#22423=CARTESIAN_POINT('Ctrl Pts',(-2.55629759922068,-0.188789295620503,
6.01121642757463));
#22424=CARTESIAN_POINT('Ctrl Pts',(-2.56027054474607,-0.251686882549192,
6.04865057572677));
#22425=CARTESIAN_POINT('Ctrl Pts',(-2.56424349027146,-0.301785308483965,
6.09885424668315));
#22426=CARTESIAN_POINT('Ctrl Pts',(-2.56821643579686,-0.351883734418738,
6.14905791763954));
#22427=CARTESIAN_POINT('Ctrl Pts',(-2.57218938132225,-0.389182999359593,
6.21203111140016));
#22428=CARTESIAN_POINT('Ctrl Pts',(-2.57616232684764,-0.409128604357937,
6.28009503442026));
#22429=CARTESIAN_POINT('Ctrl Pts',(-2.58013527237303,-0.429074209356281,
6.34815895744036));
#22430=CARTESIAN_POINT('Ctrl Pts',(-2.58410821789843,-0.431666154412113,
6.42131360971993));
#22431=CARTESIAN_POINT('Ctrl Pts',(-2.58808116342382,-0.416588405254627,
6.49060905834863));
#22432=CARTESIAN_POINT('Ctrl Pts',(-2.59205410894921,-0.401510656097141,
6.55990450697734));
#22433=CARTESIAN_POINT('Ctrl Pts',(-2.59602705447461,-0.368763212726337,
6.62534075195518));
#22434=CARTESIAN_POINT('Ctrl Pts',(-2.6,-0.322335278395778,6.67898325810255));
#22435=CARTESIAN_POINT('',(-2.6,0.322364416527282,6.67900379523473));
#22436=CARTESIAN_POINT('Origin',(-2.6,0.,6.4));
#22437=CARTESIAN_POINT('Ctrl Pts',(-2.6,0.322364416527282,6.67900379523473));
#22438=CARTESIAN_POINT('Ctrl Pts',(-2.59622409987445,0.278227326350059,
6.7299532665394));
#22439=CARTESIAN_POINT('Ctrl Pts',(-2.5924481997489,0.221801779901377,6.77028569095882));
#22440=CARTESIAN_POINT('Ctrl Pts',(-2.58867229962336,0.159274815469995,
6.79546821970908));
#22441=CARTESIAN_POINT('Ctrl Pts',(-2.58469935409796,0.0934848805420922,
6.8219648990676));
#22442=CARTESIAN_POINT('Ctrl Pts',(-2.58072640857257,0.0209401066261879,
6.83168923038829));
#22443=CARTESIAN_POINT('Ctrl Pts',(-2.57675346304718,-0.0495052156044451,
6.82345364573744));
#22444=CARTESIAN_POINT('Ctrl Pts',(-2.57278051752178,-0.119950537835078,
6.81521806108658));
#22445=CARTESIAN_POINT('Ctrl Pts',(-2.56880757199639,-0.18829640838044,
6.78902256046417));
#22446=CARTESIAN_POINT('Ctrl Pts',(-2.564834626471,-0.246200230888236,6.74806486065615));
#22447=CARTESIAN_POINT('Ctrl Pts',(-2.5608616809456,-0.304104053396033,
6.70710716084812));
#22448=CARTESIAN_POINT('Ctrl Pts',(-2.55688873542021,-0.351565827866263,
6.65138726185447));
#22449=CARTESIAN_POINT('Ctrl Pts',(-2.55291578989482,-0.382792466430557,
6.58770623363867));
#22450=CARTESIAN_POINT('Ctrl Pts',(-2.54894284436942,-0.414019104994851,
6.52402520542287));
#22451=CARTESIAN_POINT('Ctrl Pts',(-2.54496989884403,-0.429010607653208,
6.45238304798492));
#22452=CARTESIAN_POINT('Ctrl Pts',(-2.54099695331864,-0.425937046871258,
6.3815245022355));
#22453=CARTESIAN_POINT('Ctrl Pts',(-2.53702400779324,-0.422863486089309,
6.31066595648609));
#22454=CARTESIAN_POINT('Ctrl Pts',(-2.53305106226785,-0.401724861867054,
6.24059102242521));
#22455=CARTESIAN_POINT('Ctrl Pts',(-2.52907811674246,-0.36510139236472,
6.17985305598722));
#22456=CARTESIAN_POINT('Ctrl Pts',(-2.52510517121707,-0.328477922862385,
6.11911508954922));
#22457=CARTESIAN_POINT('Ctrl Pts',(-2.52113222569167,-0.276369608079971,
6.06771409073411));
#22458=CARTESIAN_POINT('Ctrl Pts',(-2.51715928016628,-0.215136804720175,
6.03192410620715));
#22459=CARTESIAN_POINT('Ctrl Pts',(-2.51318633464089,-0.153904001360379,
5.99613412168019));
#22460=CARTESIAN_POINT('Ctrl Pts',(-2.50921338911549,-0.0835467094232002,
5.97595515144138));
#22461=CARTESIAN_POINT('Ctrl Pts',(-2.5052404435901,-0.01265278349094,5.97385024536399));
#22462=CARTESIAN_POINT('Ctrl Pts',(-2.50126749806471,0.0582411424413201,
5.9717453392866));
#22463=CARTESIAN_POINT('Ctrl Pts',(-2.49729455253931,0.129671702368662,
5.98771449737062));
#22464=CARTESIAN_POINT('Ctrl Pts',(-2.49332160701392,0.192920046362828,
6.01980851841896));
#22465=CARTESIAN_POINT('Ctrl Pts',(-2.48934866148853,0.256168390356993,
6.05190253946729));
#22466=CARTESIAN_POINT('Ctrl Pts',(-2.48537571596313,0.311234518417982,
6.10012142347994));
#22467=CARTESIAN_POINT('Ctrl Pts',(-2.48140277043774,0.351397028106915,
6.15857954622212));
#22468=CARTESIAN_POINT('Ctrl Pts',(-2.47742982491235,0.391559537795848,
6.21703766896431));
#22469=CARTESIAN_POINT('Ctrl Pts',(-2.47345687938695,0.416818429112726,
6.28573503043603));
#22470=CARTESIAN_POINT('Ctrl Pts',(-2.46948393386156,0.424090588766216,
6.35628639435329));
#22471=CARTESIAN_POINT('Ctrl Pts',(-2.46866656688807,0.425586713766852,
6.37080115536172));
#22472=CARTESIAN_POINT('Ctrl Pts',(-2.46784919991458,0.426321529342654,
6.385394389189));
#22473=CARTESIAN_POINT('Ctrl Pts',(-2.46703183294109,0.426306423912841,
6.39998913682467));
#22474=CARTESIAN_POINT('Origin',(2.35,0.,6.4));
#22475=CARTESIAN_POINT('',(2.2079681670589,-0.426326761040182,6.40000738455106));
#22476=CARTESIAN_POINT('',(2.16703183294109,-0.426272942583651,6.39999240784429));
#22477=CARTESIAN_POINT('',(2.35,-0.4263,6.4));
#22478=CARTESIAN_POINT('',(2.1,0.402774227945242,6.53965891057542));
#22479=CARTESIAN_POINT('Ctrl Pts',(2.16703183294109,-0.426272942583651,
6.39999240784429));
#22480=CARTESIAN_POINT('Ctrl Pts',(2.16455261625436,-0.426244983352413,
6.44427071500844));
#22481=CARTESIAN_POINT('Ctrl Pts',(2.16207339956763,-0.419380394763561,
6.488557477259));
#22482=CARTESIAN_POINT('Ctrl Pts',(2.1595941828809,-0.405813684403497,6.53068600993882));
#22483=CARTESIAN_POINT('Ctrl Pts',(2.1556212373555,-0.384073026756357,6.59819699689588));
#22484=CARTESIAN_POINT('Ctrl Pts',(2.15164829183011,-0.34512127171195,6.66016563463643));
#22485=CARTESIAN_POINT('Ctrl Pts',(2.14767534630472,-0.293711532789595,
6.70902687081076));
#22486=CARTESIAN_POINT('Ctrl Pts',(2.14370240077932,-0.242301793867241,
6.75788810698509));
#22487=CARTESIAN_POINT('Ctrl Pts',(2.13972945525393,-0.178434071066939,
6.7936419415932));
#22488=CARTESIAN_POINT('Ctrl Pts',(2.13575650972854,-0.10990720362842,6.81192661575963));
#22489=CARTESIAN_POINT('Ctrl Pts',(2.13178356420314,-0.0413803361899007,
6.83021128992606));
#22490=CARTESIAN_POINT('Ctrl Pts',(2.12781061867775,0.031805675886835,6.83102680365082));
#22491=CARTESIAN_POINT('Ctrl Pts',(2.12383767315236,0.100723579247557,6.81426824831305));
#22492=CARTESIAN_POINT('Ctrl Pts',(2.11986472762697,0.169641482608279,6.79750969297527));
#22493=CARTESIAN_POINT('Ctrl Pts',(2.11589178210157,0.234291277252986,6.76317706857497));
#22494=CARTESIAN_POINT('Ctrl Pts',(2.11191883657618,0.286764012116973,6.71547162888731));
#22495=CARTESIAN_POINT('Ctrl Pts',(2.10794589105079,0.33923674698096,6.66776618919964));
#22496=CARTESIAN_POINT('Ctrl Pts',(2.10397294552539,0.379532422064226,6.60668793422461));
#22497=CARTESIAN_POINT('Ctrl Pts',(2.1,0.402774227945242,6.53965891057542));
#22498=CARTESIAN_POINT('',(2.1,0.0804421690761202,5.98132232055468));
#22499=CARTESIAN_POINT('Origin',(2.1,0.,6.4));
#22500=CARTESIAN_POINT('Ctrl Pts',(2.1,0.0804421690761202,5.98132232055468));
#22501=CARTESIAN_POINT('Ctrl Pts',(2.10377590012555,0.14663424989577,5.99407142716487));
#22502=CARTESIAN_POINT('Ctrl Pts',(2.1075518002511,0.209775930044154,6.02277117104005));
#22503=CARTESIAN_POINT('Ctrl Pts',(2.11132770037664,0.262848123123102,6.06432984686491));
#22504=CARTESIAN_POINT('Ctrl Pts',(2.11530064590204,0.318689889325856,6.10805726275774));
#22505=CARTESIAN_POINT('Ctrl Pts',(2.11927359142743,0.363383793828482,6.16602071609696));
#22506=CARTESIAN_POINT('Ctrl Pts',(2.12324653695282,0.391474229567156,6.2311459484684));
#22507=CARTESIAN_POINT('Ctrl Pts',(2.12721948247822,0.41956466530583,6.29627118083984));
#22508=CARTESIAN_POINT('Ctrl Pts',(2.13119242800361,0.431051632280552,6.36855819224351));
#22509=CARTESIAN_POINT('Ctrl Pts',(2.135165373529,0.4245331350138,6.43918322464256));
#22510=CARTESIAN_POINT('Ctrl Pts',(2.1391383190544,0.418014637747048,6.50980825704162));
#22511=CARTESIAN_POINT('Ctrl Pts',(2.14311126457979,0.393490676238824,6.57877131043605));
#22512=CARTESIAN_POINT('Ctrl Pts',(2.14708421010518,0.353954606539213,6.63765488796442));
#22513=CARTESIAN_POINT('Ctrl Pts',(2.15105715563058,0.314418536839601,6.69653846549279));
#22514=CARTESIAN_POINT('Ctrl Pts',(2.15503010115597,0.259870358948601,6.74534256715509));
#22515=CARTESIAN_POINT('Ctrl Pts',(2.15900304668136,0.196968276722384,6.77811005889651));
#22516=CARTESIAN_POINT('Ctrl Pts',(2.16297599220675,0.134066194496165,6.81087755063794));
#22517=CARTESIAN_POINT('Ctrl Pts',(2.16694893773215,0.0628102079347276,
6.8276084324585));
#22518=CARTESIAN_POINT('Ctrl Pts',(2.17092188325754,-0.00810215006175566,
6.82626056070251));
#22519=CARTESIAN_POINT('Ctrl Pts',(2.17489482878293,-0.0790145080582389,
6.82491268894653));
#22520=CARTESIAN_POINT('Ctrl Pts',(2.17886777430833,-0.149583237489768,
6.805486063614));
#22521=CARTESIAN_POINT('Ctrl Pts',(2.18284071983372,-0.211194676111135,
6.77035189196174));
#22522=CARTESIAN_POINT('Ctrl Pts',(2.18681366535911,-0.272806114732501,
6.73521772030948));
#22523=CARTESIAN_POINT('Ctrl Pts',(2.19078661088451,-0.325460262543706,
6.68437600233748));
#22524=CARTESIAN_POINT('Ctrl Pts',(2.1947595564099,-0.362730128342859,6.62403251342481));
#22525=CARTESIAN_POINT('Ctrl Pts',(2.19873250193529,-0.399999994142011,
6.56368902451214));
#22526=CARTESIAN_POINT('Ctrl Pts',(2.20270544746069,-0.421885577929111,
6.4938437646588));
#22527=CARTESIAN_POINT('Ctrl Pts',(2.20667839298608,-0.425715512458415,
6.42302208016789));
#22528=CARTESIAN_POINT('Ctrl Pts',(2.20710831767702,-0.426129961488313,
6.41535824722023));
#22529=CARTESIAN_POINT('Ctrl Pts',(2.20753824236796,-0.426332977570519,
6.40768298027005));
#22530=CARTESIAN_POINT('Ctrl Pts',(2.2079681670589,-0.426326761040182,6.40000738455106));
#22531=CARTESIAN_POINT('Origin',(2.35,0.,6.4));
#22532=CARTESIAN_POINT('',(2.3579681670589,-0.426284649716722,6.39998978457651));
#22533=CARTESIAN_POINT('',(2.31703183294109,-0.426305653513777,6.40001091236462));
#22534=CARTESIAN_POINT('',(2.35,-0.4263,6.4));
#22535=CARTESIAN_POINT('Ctrl Pts',(2.31703183294109,-0.426305653513777,
6.40001091236462));
#22536=CARTESIAN_POINT('Ctrl Pts',(2.31620090808447,-0.426321019141741,
6.41484782419694));
#22537=CARTESIAN_POINT('Ctrl Pts',(2.31536998322785,-0.425561575912188,
6.42968317075982));
#22538=CARTESIAN_POINT('Ctrl Pts',(2.31453905837123,-0.42401549701117,6.44443607928542));
#22539=CARTESIAN_POINT('Ctrl Pts',(2.31056611284584,-0.416623147146128,
6.51497495105736));
#22540=CARTESIAN_POINT('Ctrl Pts',(2.30659316732044,-0.391247250234886,
6.58362917867256));
#22541=CARTESIAN_POINT('Ctrl Pts',(2.30262022179505,-0.350985201969758,
6.6420187902307));
#22542=CARTESIAN_POINT('Ctrl Pts',(2.29864727626966,-0.310723153704629,
6.70040840178883));
#22543=CARTESIAN_POINT('Ctrl Pts',(2.29467433074426,-0.255574954085614,
6.74853339728991));
#22544=CARTESIAN_POINT('Ctrl Pts',(2.29070138521887,-0.192272021883084,
6.78051961378245));
#22545=CARTESIAN_POINT('Ctrl Pts',(2.28672843969348,-0.128969089680553,
6.81250583027498));
#22546=CARTESIAN_POINT('Ctrl Pts',(2.28275549416808,-0.0575114248945075,
6.82835326775898));
#22547=CARTESIAN_POINT('Ctrl Pts',(2.27878254864269,0.013378811171034,6.82612757973448));
#22548=CARTESIAN_POINT('Ctrl Pts',(2.2748096031173,0.0842690472365756,6.82390189170998));
#22549=CARTESIAN_POINT('Ctrl Pts',(2.27083665759191,0.154591854581613,6.80360307817698));
#22550=CARTESIAN_POINT('Ctrl Pts',(2.26686371206651,0.215763594163553,6.76770882270937));
#22551=CARTESIAN_POINT('Ctrl Pts',(2.26289076654112,0.276935333745493,6.73181456724177));
#22552=CARTESIAN_POINT('Ctrl Pts',(2.25891782101573,0.328956005564335,6.68032486983957));
#22553=CARTESIAN_POINT('Ctrl Pts',(2.25494487549033,0.365475937036552,6.61952459179481));
#22554=CARTESIAN_POINT('Ctrl Pts',(2.25097192996494,0.401995868508769,6.55872431375006));
#22555=CARTESIAN_POINT('Ctrl Pts',(2.24699898443955,0.423015059634361,6.48861345506275));
#22556=CARTESIAN_POINT('Ctrl Pts',(2.24302603891415,0.425967899647639,6.4177497824262));
#22557=CARTESIAN_POINT('Ctrl Pts',(2.23905309338876,0.428920739660916,6.34688610978966));
#22558=CARTESIAN_POINT('Ctrl Pts',(2.23508014786337,0.413807228561879,6.27526962320388));
#22559=CARTESIAN_POINT('Ctrl Pts',(2.23110720233797,0.382472123166929,6.21164187477894));
#22560=CARTESIAN_POINT('Ctrl Pts',(2.22713425681258,0.35113701777198,6.14801412635401));
#22561=CARTESIAN_POINT('Ctrl Pts',(2.22316131128719,0.303580318081118,6.09237511608992));
#22562=CARTESIAN_POINT('Ctrl Pts',(2.2191883657618,0.245606834378852,6.05151616024381));
#22563=CARTESIAN_POINT('Ctrl Pts',(2.2152154202364,0.187633350676587,6.0106572043977));
#22564=CARTESIAN_POINT('Ctrl Pts',(2.21124247471101,0.119243082962917,5.98457830296956));
#22565=CARTESIAN_POINT('Ctrl Pts',(2.20726952918561,0.0487837540878456,
5.97646268493538));
#22566=CARTESIAN_POINT('Ctrl Pts',(2.20329658366022,-0.0216755747872263,
5.96834706690119));
#22567=CARTESIAN_POINT('Ctrl Pts',(2.19932363813483,-0.0942039648236993,
5.97819473226094));
#22568=CARTESIAN_POINT('Ctrl Pts',(2.19535069260944,-0.159948497199684,
6.00480361749332));
#22569=CARTESIAN_POINT('Ctrl Pts',(2.19137774708404,-0.225693029575669,
6.03141250272569));
#22570=CARTESIAN_POINT('Ctrl Pts',(2.18740480155865,-0.284653704291167,
6.07478260783069));
#22571=CARTESIAN_POINT('Ctrl Pts',(2.18343185603326,-0.329633888906202,
6.12962026666635));
#22572=CARTESIAN_POINT('Ctrl Pts',(2.17945891050786,-0.374614073521237,
6.184457925502));
#22573=CARTESIAN_POINT('Ctrl Pts',(2.17548596498247,-0.40561376803581,6.25076313806833));
#22574=CARTESIAN_POINT('Ctrl Pts',(2.17151301945708,-0.41884883516816,6.32044241243827));
#22575=CARTESIAN_POINT('Ctrl Pts',(2.17001929061842,-0.423824891681104,
6.34664008892744));
#22576=CARTESIAN_POINT('Ctrl Pts',(2.16852556177975,-0.426289788029324,
6.37331471375964));
#22577=CARTESIAN_POINT('Ctrl Pts',(2.16703183294109,-0.426272942583651,
6.39999240784429));
#22578=CARTESIAN_POINT('Ctrl Pts',(2.2079681670589,-0.426326761040182,6.40000738455106));
#22579=CARTESIAN_POINT('Ctrl Pts',(2.21151118789336,-0.426275530448026,
6.3367525956958));
#22580=CARTESIAN_POINT('Ctrl Pts',(2.21505420872781,-0.412014367364063,
6.27347547866508));
#22581=CARTESIAN_POINT('Ctrl Pts',(2.21859722956226,-0.384774767183445,
6.21639147031607));
#22582=CARTESIAN_POINT('Ctrl Pts',(2.22257017508765,-0.354229802107662,
6.15238065408364));
#22583=CARTESIAN_POINT('Ctrl Pts',(2.22654312061304,-0.307365586684588,
6.09615713074728));
#22584=CARTESIAN_POINT('Ctrl Pts',(2.23051606613844,-0.249902392017012,
6.05458357301381));
#22585=CARTESIAN_POINT('Ctrl Pts',(2.23448901166383,-0.192439197349434,
6.01301001528034));
#22586=CARTESIAN_POINT('Ctrl Pts',(2.23846195718922,-0.124377023437354,
5.98608642314976));
#22587=CARTESIAN_POINT('Ctrl Pts',(2.24243490271462,-0.0540235759521597,
5.97709910512957));
#22588=CARTESIAN_POINT('Ctrl Pts',(2.24640784824001,0.0163298715330345,
5.96811178710938));
#22589=CARTESIAN_POINT('Ctrl Pts',(2.2503807937654,0.0889745925913431,5.97706074319959));
#22590=CARTESIAN_POINT('Ctrl Pts',(2.2543537392908,0.155043533545503,6.00285365883444));
#22591=CARTESIAN_POINT('Ctrl Pts',(2.25832668481619,0.221112474499663,6.02864657446929));
#22592=CARTESIAN_POINT('Ctrl Pts',(2.26229963034158,0.280605635349674,6.07128344964878));
#22593=CARTESIAN_POINT('Ctrl Pts',(2.26627257586698,0.326261248855651,6.1255600045331));
#22594=CARTESIAN_POINT('Ctrl Pts',(2.27024552139237,0.371916862361629,6.17983655941743));
#22595=CARTESIAN_POINT('Ctrl Pts',(2.27421846691776,0.403734928523572,6.24575279400659));
#22596=CARTESIAN_POINT('Ctrl Pts',(2.27819141244315,0.417831717081485,6.31526293721211));
#22597=CARTESIAN_POINT('Ctrl Pts',(2.28216435796855,0.431928505639397,6.38477308041763));
#22598=CARTESIAN_POINT('Ctrl Pts',(2.28613730349394,0.42830401659328,6.45787713223949));
#22599=CARTESIAN_POINT('Ctrl Pts',(2.29011024901934,0.407400657020557,6.52565197280568));
#22600=CARTESIAN_POINT('Ctrl Pts',(2.29408319454473,0.386497297447833,6.59342681337187));
#22601=CARTESIAN_POINT('Ctrl Pts',(2.29805614007012,0.348315067348504,6.65587244268238));
#22602=CARTESIAN_POINT('Ctrl Pts',(2.30202908559551,0.297514510269819,6.70536671362482));
#22603=CARTESIAN_POINT('Ctrl Pts',(2.30600203112091,0.246713953191133,6.75486098456727));
#22604=CARTESIAN_POINT('Ctrl Pts',(2.3099749766463,0.18329506913309,6.79140389714166));
#22605=CARTESIAN_POINT('Ctrl Pts',(2.31394792217169,0.114998801196742,6.81053500378618));
#22606=CARTESIAN_POINT('Ctrl Pts',(2.31792086769709,0.0467025332603938,
6.8296661104307));
#22607=CARTESIAN_POINT('Ctrl Pts',(2.32189381322248,-0.0264711185542592,
6.83138541114536));
#22608=CARTESIAN_POINT('Ctrl Pts',(2.32586675874787,-0.0955905389447022,
6.81548304715754));
#22609=CARTESIAN_POINT('Ctrl Pts',(2.32983970427327,-0.164709959335145,
6.79958068316972));
#22610=CARTESIAN_POINT('Ctrl Pts',(2.33381264979866,-0.229775148301378,
6.76605665447942));
#22611=CARTESIAN_POINT('Ctrl Pts',(2.33778559532405,-0.282844213879021,
6.71900292206431));
#22612=CARTESIAN_POINT('Ctrl Pts',(2.34175854084945,-0.335913279456664,
6.67194918964919));
#22613=CARTESIAN_POINT('Ctrl Pts',(2.34573148637484,-0.376986221645717,
6.61136575350926));
#22614=CARTESIAN_POINT('Ctrl Pts',(2.34970443190023,-0.40104965502802,6.54464746044443));
#22615=CARTESIAN_POINT('Ctrl Pts',(2.35245901028646,-0.417733652598481,
6.49838939653));
#22616=CARTESIAN_POINT('Ctrl Pts',(2.35521358867268,-0.42624097353767,6.44918223268425));
#22617=CARTESIAN_POINT('Ctrl Pts',(2.3579681670589,-0.426284649716722,6.39998978457651));
#22618=CARTESIAN_POINT('Origin',(2.35,0.,6.4));
#22619=CARTESIAN_POINT('',(2.50796816705891,-0.426290360635438,6.40001083203199));
#22620=CARTESIAN_POINT('',(2.46703183294109,-0.426306423912841,6.39998913682467));
#22621=CARTESIAN_POINT('',(2.35,-0.4263,6.4));
#22622=CARTESIAN_POINT('',(2.6,0.32233527839578,6.67898325810255));
#22623=CARTESIAN_POINT('Ctrl Pts',(2.50796816705891,-0.426290360635438,
6.40001083203199));
#22624=CARTESIAN_POINT('Ctrl Pts',(2.51083482602818,-0.426241188929821,
6.34881879719149));
#22625=CARTESIAN_POINT('Ctrl Pts',(2.51370148499746,-0.417011809736389,
6.29760951317986));
#22626=CARTESIAN_POINT('Ctrl Pts',(2.51656814396674,-0.398972669717071,
6.24971854193924));
#22627=CARTESIAN_POINT('Ctrl Pts',(2.52054108949214,-0.373971955858283,
6.18334572887142));
#22628=CARTESIAN_POINT('Ctrl Pts',(2.52451403501753,-0.332049803576913,
6.12334659907732));
#22629=CARTESIAN_POINT('Ctrl Pts',(2.52848698054292,-0.278323314671085,
6.07704505632467));
#22630=CARTESIAN_POINT('Ctrl Pts',(2.53245992606832,-0.224596825765257,
6.03074351357203));
#22631=CARTESIAN_POINT('Ctrl Pts',(2.53643287159371,-0.159066000234972,
5.99813955786084));
#22632=CARTESIAN_POINT('Ctrl Pts',(2.5404058171191,-0.089729440237079,5.98321202621739));
#22633=CARTESIAN_POINT('Ctrl Pts',(2.5443787626445,-0.0203928802391868,
5.96828449457393));
#22634=CARTESIAN_POINT('Ctrl Pts',(2.54835170816989,0.0527494142263132,
5.97103338699821));
#22635=CARTESIAN_POINT('Ctrl Pts',(2.55232465369528,0.120769354923407,5.99112490728642));
#22636=CARTESIAN_POINT('Ctrl Pts',(2.55629759922068,0.188789295620503,6.01121642757463));
#22637=CARTESIAN_POINT('Ctrl Pts',(2.56027054474607,0.251686882549192,6.04865057572677));
#22638=CARTESIAN_POINT('Ctrl Pts',(2.56424349027146,0.301785308483965,6.09885424668315));
#22639=CARTESIAN_POINT('Ctrl Pts',(2.56821643579686,0.351883734418738,6.14905791763954));
#22640=CARTESIAN_POINT('Ctrl Pts',(2.57218938132225,0.389182999359593,6.21203111140016));
#22641=CARTESIAN_POINT('Ctrl Pts',(2.57616232684764,0.409128604357937,6.28009503442026));
#22642=CARTESIAN_POINT('Ctrl Pts',(2.58013527237303,0.429074209356281,6.34815895744036));
#22643=CARTESIAN_POINT('Ctrl Pts',(2.58410821789843,0.431666154412113,6.42131360971993));
#22644=CARTESIAN_POINT('Ctrl Pts',(2.58808116342382,0.416588405254627,6.49060905834863));
#22645=CARTESIAN_POINT('Ctrl Pts',(2.59205410894921,0.401510656097141,6.55990450697734));
#22646=CARTESIAN_POINT('Ctrl Pts',(2.59602705447461,0.368763212726337,6.62534075195518));
#22647=CARTESIAN_POINT('Ctrl Pts',(2.6,0.322335278395778,6.67898325810255));
#22648=CARTESIAN_POINT('',(2.6,-0.322364416527282,6.67900379523473));
#22649=CARTESIAN_POINT('Origin',(2.6,0.,6.4));
#22650=CARTESIAN_POINT('Ctrl Pts',(2.6,-0.322364416527282,6.67900379523473));
#22651=CARTESIAN_POINT('Ctrl Pts',(2.59622409987445,-0.278227326350059,
6.7299532665394));
#22652=CARTESIAN_POINT('Ctrl Pts',(2.5924481997489,-0.221801779901377,6.77028569095882));
#22653=CARTESIAN_POINT('Ctrl Pts',(2.58867229962336,-0.159274815469995,
6.79546821970908));
#22654=CARTESIAN_POINT('Ctrl Pts',(2.58469935409796,-0.0934848805420922,
6.8219648990676));
#22655=CARTESIAN_POINT('Ctrl Pts',(2.58072640857257,-0.0209401066261879,
6.83168923038829));
#22656=CARTESIAN_POINT('Ctrl Pts',(2.57675346304718,0.0495052156044451,
6.82345364573744));
#22657=CARTESIAN_POINT('Ctrl Pts',(2.57278051752178,0.119950537835078,6.81521806108658));
#22658=CARTESIAN_POINT('Ctrl Pts',(2.56880757199639,0.18829640838044,6.78902256046417));
#22659=CARTESIAN_POINT('Ctrl Pts',(2.564834626471,0.246200230888236,6.74806486065615));
#22660=CARTESIAN_POINT('Ctrl Pts',(2.5608616809456,0.304104053396033,6.70710716084812));
#22661=CARTESIAN_POINT('Ctrl Pts',(2.55688873542021,0.351565827866263,6.65138726185447));
#22662=CARTESIAN_POINT('Ctrl Pts',(2.55291578989482,0.382792466430557,6.58770623363867));
#22663=CARTESIAN_POINT('Ctrl Pts',(2.54894284436942,0.414019104994851,6.52402520542287));
#22664=CARTESIAN_POINT('Ctrl Pts',(2.54496989884403,0.429010607653208,6.45238304798492));
#22665=CARTESIAN_POINT('Ctrl Pts',(2.54099695331864,0.425937046871258,6.3815245022355));
#22666=CARTESIAN_POINT('Ctrl Pts',(2.53702400779324,0.422863486089309,6.31066595648609));
#22667=CARTESIAN_POINT('Ctrl Pts',(2.53305106226785,0.401724861867054,6.24059102242521));
#22668=CARTESIAN_POINT('Ctrl Pts',(2.52907811674246,0.36510139236472,6.17985305598722));
#22669=CARTESIAN_POINT('Ctrl Pts',(2.52510517121707,0.328477922862385,6.11911508954922));
#22670=CARTESIAN_POINT('Ctrl Pts',(2.52113222569167,0.276369608079971,6.06771409073411));
#22671=CARTESIAN_POINT('Ctrl Pts',(2.51715928016628,0.215136804720175,6.03192410620715));
#22672=CARTESIAN_POINT('Ctrl Pts',(2.51318633464089,0.153904001360379,5.99613412168019));
#22673=CARTESIAN_POINT('Ctrl Pts',(2.50921338911549,0.0835467094232002,
5.97595515144138));
#22674=CARTESIAN_POINT('Ctrl Pts',(2.5052404435901,0.01265278349094,5.97385024536399));
#22675=CARTESIAN_POINT('Ctrl Pts',(2.50126749806471,-0.0582411424413201,
5.9717453392866));
#22676=CARTESIAN_POINT('Ctrl Pts',(2.49729455253931,-0.129671702368662,
5.98771449737062));
#22677=CARTESIAN_POINT('Ctrl Pts',(2.49332160701392,-0.192920046362828,
6.01980851841896));
#22678=CARTESIAN_POINT('Ctrl Pts',(2.48934866148853,-0.256168390356993,
6.05190253946729));
#22679=CARTESIAN_POINT('Ctrl Pts',(2.48537571596313,-0.311234518417982,
6.10012142347994));
#22680=CARTESIAN_POINT('Ctrl Pts',(2.48140277043774,-0.351397028106915,
6.15857954622212));
#22681=CARTESIAN_POINT('Ctrl Pts',(2.47742982491235,-0.391559537795848,
6.21703766896431));
#22682=CARTESIAN_POINT('Ctrl Pts',(2.47345687938695,-0.416818429112726,
6.28573503043603));
#22683=CARTESIAN_POINT('Ctrl Pts',(2.46948393386156,-0.424090588766216,
6.35628639435329));
#22684=CARTESIAN_POINT('Ctrl Pts',(2.46866656688807,-0.425586713766852,
6.37080115536172));
#22685=CARTESIAN_POINT('Ctrl Pts',(2.46784919991458,-0.426321529342654,
6.385394389189));
#22686=CARTESIAN_POINT('Ctrl Pts',(2.46703183294109,-0.426306423912841,
6.39998913682467));
#22687=CARTESIAN_POINT('Origin',(-2.93123464956316,0.,6.4));
#22688=CARTESIAN_POINT('',(-2.11876535043684,0.509867636461186,6.39999091897679));
#22689=CARTESIAN_POINT('',(-2.10623464956316,0.509830151085518,6.39998162138192));
#22690=CARTESIAN_POINT('',(-2.93123464956316,0.5099,6.4));
#22691=CARTESIAN_POINT('',(-2.1,0.492610334572591,6.53165511107542));
#22692=CARTESIAN_POINT('Ctrl Pts',(-2.10623464956316,0.509830060291024,
6.39998159749211));
#22693=CARTESIAN_POINT('Ctrl Pts',(-2.1041564330421,0.509817985963964,6.44437440316355));
#22694=CARTESIAN_POINT('Ctrl Pts',(-2.10207821652105,0.504071192426059,
6.48877233215731));
#22695=CARTESIAN_POINT('Ctrl Pts',(-2.1,0.492610334572592,6.53165511107541));
#22696=CARTESIAN_POINT('',(-2.1,0.360348823959177,6.76081852140067));
#22697=CARTESIAN_POINT('Origin',(-2.1,0.,6.4));
#22698=CARTESIAN_POINT('Ctrl Pts',(-2.11876535043684,0.509867636461186,
6.39999091897678));
#22699=CARTESIAN_POINT('Ctrl Pts',(-2.11628613375011,0.509834194256146,
6.45295246911284));
#22700=CARTESIAN_POINT('Ctrl Pts',(-2.11003101693783,0.489118231027634,
6.58660111045784));
#22701=CARTESIAN_POINT('Ctrl Pts',(-2.10377590012555,0.417372467378852,
6.70381704168278));
#22702=CARTESIAN_POINT('Ctrl Pts',(-2.1,0.360348823959177,6.76081852140067));
#22703=CARTESIAN_POINT('Origin',(-2.93123464956316,0.,6.4));
#22704=CARTESIAN_POINT('',(-2.26876535043684,0.509906762201912,6.4000130523451));
#22705=CARTESIAN_POINT('',(-2.25623464956316,0.509932009041494,6.40000883270604));
#22706=CARTESIAN_POINT('',(-2.93123464956316,0.5099,6.4));
#22707=CARTESIAN_POINT('Ctrl Pts',(-2.25623464956316,0.509932009041494,
6.40000883270604));
#22708=CARTESIAN_POINT('Ctrl Pts',(-2.25580472487222,0.509939444670906,
6.40918965901876));
#22709=CARTESIAN_POINT('Ctrl Pts',(-2.25140185465588,0.507452628870696,
6.50320671872761));
#22710=CARTESIAN_POINT('Ctrl Pts',(-2.24302603891415,0.45226492573298,6.67933176541862));
#22711=CARTESIAN_POINT('Ctrl Pts',(-2.23110720233797,0.263325094846747,
6.86176802153349));
#22712=CARTESIAN_POINT('Ctrl Pts',(-2.2191883657618,0.0101020467317839,
6.93147693256131));
#22713=CARTESIAN_POINT('Ctrl Pts',(-2.20726952918561,-0.245587098572064,
6.87144120673232));
#22714=CARTESIAN_POINT('Ctrl Pts',(-2.19535069260943,-0.441323311848774,
6.69631656607358));
#22715=CARTESIAN_POINT('Ctrl Pts',(-2.18343185603326,-0.529323086465549,
6.44885519432254));
#22716=CARTESIAN_POINT('Ctrl Pts',(-2.17151301945708,-0.488104195118536,
6.18946640393034));
#22717=CARTESIAN_POINT('Ctrl Pts',(-2.1595941828809,-0.327728249264285,
5.98147509599461));
#22718=CARTESIAN_POINT('Ctrl Pts',(-2.14767534630472,-0.0873481558956701,
5.87565064933844));
#22719=CARTESIAN_POINT('Ctrl Pts',(-2.13575650972854,0.174357740366956,
5.89783918404992));
#22720=CARTESIAN_POINT('Ctrl Pts',(-2.12383767315236,0.393492635182685,
6.04259742479108));
#22721=CARTESIAN_POINT('Ctrl Pts',(-2.11399705309723,0.495113210733723,
6.23418199944647));
#22722=CARTESIAN_POINT('Ctrl Pts',(-2.1081293785675,0.509841068565406,6.35950827065745));
#22723=CARTESIAN_POINT('Ctrl Pts',(-2.10623464956316,0.509830060291024,
6.39998159749211));
#22724=CARTESIAN_POINT('Ctrl Pts',(-2.26876535043684,0.509906762201912,
6.4000130523451));
#22725=CARTESIAN_POINT('Ctrl Pts',(-2.26793442558022,0.509925141122153,
6.41775957203382));
#22726=CARTESIAN_POINT('Ctrl Pts',(-2.2631305551982,0.504673506244106,6.52034765288796));
#22727=CARTESIAN_POINT('Ctrl Pts',(-2.2543537392908,0.437620931409163,6.70175770318116));
#22728=CARTESIAN_POINT('Ctrl Pts',(-2.24243490271462,0.239731649313908,
6.87444549491937));
#22729=CARTESIAN_POINT('Ctrl Pts',(-2.23051606613844,-0.0166811816108265,
6.93131114145764));
#22730=CARTESIAN_POINT('Ctrl Pts',(-2.21859722956226,-0.269021783055123,
6.85847254173578));
#22731=CARTESIAN_POINT('Ctrl Pts',(-2.20667839298608,-0.455688500581004,
6.67371112931225));
#22732=CARTESIAN_POINT('Ctrl Pts',(-2.1947595564099,-0.53111204424701,6.42213106706975));
#22733=CARTESIAN_POINT('Ctrl Pts',(-2.18284071983372,-0.476879959029563,
6.1651483330086));
#22734=CARTESIAN_POINT('Ctrl Pts',(-2.17092188325754,-0.306231393425269,
5.96549786619889));
#22735=CARTESIAN_POINT('Ctrl Pts',(-2.15900304668136,-0.0608253588918372,
5.8719184725451));
#22736=CARTESIAN_POINT('Ctrl Pts',(-2.14708421010518,0.199429574813985,
5.90725502825896));
#22737=CARTESIAN_POINT('Ctrl Pts',(-2.135165373529,0.410999230249818,6.06288076079265));
#22738=CARTESIAN_POINT('Ctrl Pts',(-2.12572575363955,0.49909782676439,6.25131475216463));
#22739=CARTESIAN_POINT('Ctrl Pts',(-2.1202590792755,0.50988778540031,6.36808156825251));
#22740=CARTESIAN_POINT('Ctrl Pts',(-2.11876535043684,0.509867636461186,
6.39999091897678));
#22741=CARTESIAN_POINT('Origin',(-2.93123464956316,0.,6.4));
#22742=CARTESIAN_POINT('',(-2.41876535043684,0.509907683680876,6.39998700649049));
#22743=CARTESIAN_POINT('',(-2.40623464956316,0.509881639433629,6.39998778127036));
#22744=CARTESIAN_POINT('',(-2.93123464956316,0.5099,6.4));
#22745=CARTESIAN_POINT('Ctrl Pts',(-2.40623464956316,0.509881639433629,
6.39998778127036));
#22746=CARTESIAN_POINT('Ctrl Pts',(-2.40348007117693,0.50982939809256,6.45882716501453));
#22747=CARTESIAN_POINT('Ctrl Pts',(-2.39675254726532,0.484977325655459,
6.60257394605883));
#22748=CARTESIAN_POINT('Ctrl Pts',(-2.38605207782831,0.352660304885654,
6.79774427841866));
#22749=CARTESIAN_POINT('Ctrl Pts',(-2.37413324125213,0.11918571055855,6.91803915687878));
#22750=CARTESIAN_POINT('Ctrl Pts',(-2.36221440467595,-0.143384627656033,
6.91186975902934));
#22751=CARTESIAN_POINT('Ctrl Pts',(-2.35029556809977,-0.370951756306248,
6.78074216492885));
#22752=CARTESIAN_POINT('Ctrl Pts',(-2.33837673152359,-0.507961743129952,
6.55666738389136));
#22753=CARTESIAN_POINT('Ctrl Pts',(-2.32645789494741,-0.520967562726117,
6.29434679258967));
#22754=CARTESIAN_POINT('Ctrl Pts',(-2.31453905837123,-0.406794220460285,
6.05781837586191));
#22755=CARTESIAN_POINT('Ctrl Pts',(-2.30262022179505,-0.193313835397505,
5.904823705531));
#22756=CARTESIAN_POINT('Ctrl Pts',(-2.29070138521887,0.067358531017915,
5.872712004543));
#22757=CARTESIAN_POINT('Ctrl Pts',(-2.27878254864269,0.311587260629241,
5.96932241712133));
#22758=CARTESIAN_POINT('Ctrl Pts',(-2.26729363675745,0.473685134411606,
6.16379304907585));
#22759=CARTESIAN_POINT('Ctrl Pts',(-2.25977767039761,0.509870731821366,
6.32434939841728));
#22760=CARTESIAN_POINT('Ctrl Pts',(-2.25623464956316,0.509932009041494,
6.40000883270604));
#22761=CARTESIAN_POINT('Ctrl Pts',(-2.41876535043684,0.509907683680876,
6.3999870064905));
#22762=CARTESIAN_POINT('Ctrl Pts',(-2.41560977188494,0.509837930394076,
6.46738208429797));
#22763=CARTESIAN_POINT('Ctrl Pts',(-2.40848124780764,0.479478777569272,
6.61969007117178));
#22764=CARTESIAN_POINT('Ctrl Pts',(-2.39737977820495,0.332178326477852,
6.81500283186379));
#22765=CARTESIAN_POINT('Ctrl Pts',(-2.38546094162877,0.092940867251264,
6.92338493135519));
#22766=CARTESIAN_POINT('Ctrl Pts',(-2.37354210505259,-0.168985416607936,
6.90399773818908));
#22767=CARTESIAN_POINT('Ctrl Pts',(-2.36162326847641,-0.38965879870384,
6.76157407502307));
#22768=CARTESIAN_POINT('Ctrl Pts',(-2.34970443190023,-0.515208255680234,
6.5308825596382));
#22769=CARTESIAN_POINT('Ctrl Pts',(-2.33778559532405,-0.514984518987432,
6.26823985300105));
#22770=CARTESIAN_POINT('Ctrl Pts',(-2.32586675874787,-0.389042207488899,
6.03776257519368));
#22771=CARTESIAN_POINT('Ctrl Pts',(-2.31394792217169,-0.168126493747137,
5.89571508724314));
#22772=CARTESIAN_POINT('Ctrl Pts',(-2.30202908559551,0.0938324405162212,
5.87677417471489));
#22773=CARTESIAN_POINT('Ctrl Pts',(-2.29011024901934,0.332884898468083,
5.98556371357228));
#22774=CARTESIAN_POINT('Ctrl Pts',(-2.27902233729978,0.479672887909896,
6.18088831601448));
#22775=CARTESIAN_POINT('Ctrl Pts',(-2.27190737110561,0.50983726500634,6.33290718685512));
#22776=CARTESIAN_POINT('Ctrl Pts',(-2.26876535043684,0.509906762201912,
6.4000130523451));
#22777=CARTESIAN_POINT('Origin',(-2.93123464956316,0.,6.4));
#22778=CARTESIAN_POINT('',(-2.56876535043684,0.509867809550215,6.40001069114481));
#22779=CARTESIAN_POINT('',(-2.55623464956316,0.509888470297935,6.40001295625876));
#22780=CARTESIAN_POINT('',(-2.93123464956316,0.5099,6.4));
#22781=CARTESIAN_POINT('',(-2.6,0.132288496556896,5.90755938055567));
#22782=CARTESIAN_POINT('Ctrl Pts',(-2.6,0.132288496556895,5.90755938055567));
#22783=CARTESIAN_POINT('Ctrl Pts',(-2.59602705447461,0.214239653399634,
5.92957461427473));
#22784=CARTESIAN_POINT('Ctrl Pts',(-2.58808116342382,0.366850103542102,
6.0153123398751));
#22785=CARTESIAN_POINT('Ctrl Pts',(-2.57766961356943,0.488635125282487,
6.20977428615126));
#22786=CARTESIAN_POINT('Ctrl Pts',(-2.57123100924044,0.509836321405008,
6.34733983573258));
#22787=CARTESIAN_POINT('Ctrl Pts',(-2.56876535043684,0.509867809550215,
6.40001069114481));
#22788=CARTESIAN_POINT('',(-2.6,-0.132303594671782,5.90751949357016));
#22789=CARTESIAN_POINT('Origin',(-2.6,0.,6.4));
#22790=CARTESIAN_POINT('Ctrl Pts',(-2.6,-0.132303594671782,5.90751949357016));
#22791=CARTESIAN_POINT('Ctrl Pts',(-2.59622409987445,-0.0544270437755129,
5.88663631098165));
#22792=CARTESIAN_POINT('Ctrl Pts',(-2.58847525422351,0.115765473878103,
5.88226868015152));
#22793=CARTESIAN_POINT('Ctrl Pts',(-2.57675346304718,0.347023432783479,
5.99732787846002));
#22794=CARTESIAN_POINT('Ctrl Pts',(-2.56594091302711,0.483490786405975,
6.19264042843836));
#22795=CARTESIAN_POINT('Ctrl Pts',(-2.55910130853244,0.509829655724409,
6.3387818547688));
#22796=CARTESIAN_POINT('Ctrl Pts',(-2.55623464956316,0.509888470297935,
6.40001295625876));
#22797=CARTESIAN_POINT('Origin',(2.93123464956316,0.,6.4));
#22798=CARTESIAN_POINT('',(2.11876535043684,-0.509867636461186,6.39999091897679));
#22799=CARTESIAN_POINT('',(2.10623464956316,-0.509830151085518,6.39998162138192));
#22800=CARTESIAN_POINT('',(2.93123464956316,-0.5099,6.4));
#22801=CARTESIAN_POINT('',(2.1,-0.492610334572591,6.53165511107542));
#22802=CARTESIAN_POINT('Ctrl Pts',(2.10623464956316,-0.509830060291024,
6.39998159749211));
#22803=CARTESIAN_POINT('Ctrl Pts',(2.1041564330421,-0.509817985963964,6.44437440316355));
#22804=CARTESIAN_POINT('Ctrl Pts',(2.10207821652105,-0.504071192426059,
6.48877233215731));
#22805=CARTESIAN_POINT('Ctrl Pts',(2.1,-0.492610334572592,6.53165511107541));
#22806=CARTESIAN_POINT('',(2.1,-0.360348823959177,6.76081852140067));
#22807=CARTESIAN_POINT('Origin',(2.1,0.,6.4));
#22808=CARTESIAN_POINT('Ctrl Pts',(2.11876535043684,-0.509867636461186,
6.39999091897678));
#22809=CARTESIAN_POINT('Ctrl Pts',(2.11628613375011,-0.509834194256146,
6.45295246911284));
#22810=CARTESIAN_POINT('Ctrl Pts',(2.11003101693783,-0.489118231027634,
6.58660111045784));
#22811=CARTESIAN_POINT('Ctrl Pts',(2.10377590012555,-0.417372467378852,
6.70381704168278));
#22812=CARTESIAN_POINT('Ctrl Pts',(2.1,-0.360348823959177,6.76081852140067));
#22813=CARTESIAN_POINT('Origin',(2.93123464956316,0.,6.4));
#22814=CARTESIAN_POINT('',(2.26876535043684,-0.509906762201912,6.4000130523451));
#22815=CARTESIAN_POINT('',(2.25623464956316,-0.509932009041494,6.40000883270604));
#22816=CARTESIAN_POINT('',(2.93123464956316,-0.5099,6.4));
#22817=CARTESIAN_POINT('Ctrl Pts',(2.25623464956316,-0.509932009041494,
6.40000883270604));
#22818=CARTESIAN_POINT('Ctrl Pts',(2.25580472487222,-0.509939444670906,
6.40918965901876));
#22819=CARTESIAN_POINT('Ctrl Pts',(2.25140185465588,-0.507452628870696,
6.50320671872761));
#22820=CARTESIAN_POINT('Ctrl Pts',(2.24302603891415,-0.45226492573298,6.67933176541862));
#22821=CARTESIAN_POINT('Ctrl Pts',(2.23110720233797,-0.263325094846747,
6.86176802153349));
#22822=CARTESIAN_POINT('Ctrl Pts',(2.2191883657618,-0.0101020467317839,
6.93147693256131));
#22823=CARTESIAN_POINT('Ctrl Pts',(2.20726952918561,0.245587098572064,6.87144120673232));
#22824=CARTESIAN_POINT('Ctrl Pts',(2.19535069260943,0.441323311848774,6.69631656607358));
#22825=CARTESIAN_POINT('Ctrl Pts',(2.18343185603326,0.529323086465549,6.44885519432254));
#22826=CARTESIAN_POINT('Ctrl Pts',(2.17151301945708,0.488104195118536,6.18946640393034));
#22827=CARTESIAN_POINT('Ctrl Pts',(2.1595941828809,0.327728249264285,5.98147509599461));
#22828=CARTESIAN_POINT('Ctrl Pts',(2.14767534630472,0.0873481558956701,
5.87565064933844));
#22829=CARTESIAN_POINT('Ctrl Pts',(2.13575650972854,-0.174357740366956,
5.89783918404992));
#22830=CARTESIAN_POINT('Ctrl Pts',(2.12383767315236,-0.393492635182685,
6.04259742479108));
#22831=CARTESIAN_POINT('Ctrl Pts',(2.11399705309723,-0.495113210733723,
6.23418199944647));
#22832=CARTESIAN_POINT('Ctrl Pts',(2.1081293785675,-0.509841068565406,6.35950827065745));
#22833=CARTESIAN_POINT('Ctrl Pts',(2.10623464956316,-0.509830060291024,
6.39998159749211));
#22834=CARTESIAN_POINT('Ctrl Pts',(2.26876535043684,-0.509906762201912,
6.4000130523451));
#22835=CARTESIAN_POINT('Ctrl Pts',(2.26793442558022,-0.509925141122153,
6.41775957203382));
#22836=CARTESIAN_POINT('Ctrl Pts',(2.2631305551982,-0.504673506244106,6.52034765288796));
#22837=CARTESIAN_POINT('Ctrl Pts',(2.2543537392908,-0.437620931409163,6.70175770318116));
#22838=CARTESIAN_POINT('Ctrl Pts',(2.24243490271462,-0.239731649313908,
6.87444549491937));
#22839=CARTESIAN_POINT('Ctrl Pts',(2.23051606613844,0.0166811816108265,
6.93131114145764));
#22840=CARTESIAN_POINT('Ctrl Pts',(2.21859722956226,0.269021783055123,6.85847254173578));
#22841=CARTESIAN_POINT('Ctrl Pts',(2.20667839298608,0.455688500581004,6.67371112931225));
#22842=CARTESIAN_POINT('Ctrl Pts',(2.1947595564099,0.53111204424701,6.42213106706975));
#22843=CARTESIAN_POINT('Ctrl Pts',(2.18284071983372,0.476879959029563,6.1651483330086));
#22844=CARTESIAN_POINT('Ctrl Pts',(2.17092188325754,0.306231393425269,5.96549786619889));
#22845=CARTESIAN_POINT('Ctrl Pts',(2.15900304668136,0.0608253588918372,
5.8719184725451));
#22846=CARTESIAN_POINT('Ctrl Pts',(2.14708421010518,-0.199429574813985,
5.90725502825896));
#22847=CARTESIAN_POINT('Ctrl Pts',(2.135165373529,-0.410999230249818,6.06288076079265));
#22848=CARTESIAN_POINT('Ctrl Pts',(2.12572575363955,-0.49909782676439,6.25131475216463));
#22849=CARTESIAN_POINT('Ctrl Pts',(2.1202590792755,-0.50988778540031,6.36808156825251));
#22850=CARTESIAN_POINT('Ctrl Pts',(2.11876535043684,-0.509867636461186,
6.39999091897678));
#22851=CARTESIAN_POINT('Origin',(2.93123464956316,0.,6.4));
#22852=CARTESIAN_POINT('',(2.41876535043684,-0.509907683680876,6.39998700649049));
#22853=CARTESIAN_POINT('',(2.40623464956316,-0.509881639433629,6.39998778127036));
#22854=CARTESIAN_POINT('',(2.93123464956316,-0.5099,6.4));
#22855=CARTESIAN_POINT('Ctrl Pts',(2.40623464956316,-0.509881639433629,
6.39998778127036));
#22856=CARTESIAN_POINT('Ctrl Pts',(2.40348007117693,-0.50982939809256,6.45882716501453));
#22857=CARTESIAN_POINT('Ctrl Pts',(2.39675254726532,-0.484977325655459,
6.60257394605883));
#22858=CARTESIAN_POINT('Ctrl Pts',(2.38605207782831,-0.352660304885654,
6.79774427841866));
#22859=CARTESIAN_POINT('Ctrl Pts',(2.37413324125213,-0.11918571055855,6.91803915687878));
#22860=CARTESIAN_POINT('Ctrl Pts',(2.36221440467595,0.143384627656033,6.91186975902934));
#22861=CARTESIAN_POINT('Ctrl Pts',(2.35029556809977,0.370951756306248,6.78074216492885));
#22862=CARTESIAN_POINT('Ctrl Pts',(2.33837673152359,0.507961743129952,6.55666738389136));
#22863=CARTESIAN_POINT('Ctrl Pts',(2.32645789494741,0.520967562726117,6.29434679258967));
#22864=CARTESIAN_POINT('Ctrl Pts',(2.31453905837123,0.406794220460285,6.05781837586191));
#22865=CARTESIAN_POINT('Ctrl Pts',(2.30262022179505,0.193313835397505,5.904823705531));
#22866=CARTESIAN_POINT('Ctrl Pts',(2.29070138521887,-0.067358531017915,
5.872712004543));
#22867=CARTESIAN_POINT('Ctrl Pts',(2.27878254864269,-0.311587260629241,
5.96932241712133));
#22868=CARTESIAN_POINT('Ctrl Pts',(2.26729363675745,-0.473685134411606,
6.16379304907585));
#22869=CARTESIAN_POINT('Ctrl Pts',(2.25977767039761,-0.509870731821366,
6.32434939841728));
#22870=CARTESIAN_POINT('Ctrl Pts',(2.25623464956316,-0.509932009041494,
6.40000883270604));
#22871=CARTESIAN_POINT('Ctrl Pts',(2.41876535043684,-0.509907683680876,
6.3999870064905));
#22872=CARTESIAN_POINT('Ctrl Pts',(2.41560977188494,-0.509837930394076,
6.46738208429797));
#22873=CARTESIAN_POINT('Ctrl Pts',(2.40848124780764,-0.479478777569272,
6.61969007117178));
#22874=CARTESIAN_POINT('Ctrl Pts',(2.39737977820495,-0.332178326477852,
6.81500283186379));
#22875=CARTESIAN_POINT('Ctrl Pts',(2.38546094162877,-0.092940867251264,
6.92338493135519));
#22876=CARTESIAN_POINT('Ctrl Pts',(2.37354210505259,0.168985416607936,6.90399773818908));
#22877=CARTESIAN_POINT('Ctrl Pts',(2.36162326847641,0.38965879870384,6.76157407502307));
#22878=CARTESIAN_POINT('Ctrl Pts',(2.34970443190023,0.515208255680234,6.5308825596382));
#22879=CARTESIAN_POINT('Ctrl Pts',(2.33778559532405,0.514984518987432,6.26823985300105));
#22880=CARTESIAN_POINT('Ctrl Pts',(2.32586675874787,0.389042207488899,6.03776257519368));
#22881=CARTESIAN_POINT('Ctrl Pts',(2.31394792217169,0.168126493747137,5.89571508724314));
#22882=CARTESIAN_POINT('Ctrl Pts',(2.30202908559551,-0.0938324405162212,
5.87677417471489));
#22883=CARTESIAN_POINT('Ctrl Pts',(2.29011024901934,-0.332884898468083,
5.98556371357228));
#22884=CARTESIAN_POINT('Ctrl Pts',(2.27902233729978,-0.479672887909896,
6.18088831601448));
#22885=CARTESIAN_POINT('Ctrl Pts',(2.27190737110561,-0.50983726500634,6.33290718685512));
#22886=CARTESIAN_POINT('Ctrl Pts',(2.26876535043684,-0.509906762201912,
6.4000130523451));
#22887=CARTESIAN_POINT('Origin',(2.93123464956316,0.,6.4));
#22888=CARTESIAN_POINT('',(2.56876535043684,-0.509867809550215,6.40001069114481));
#22889=CARTESIAN_POINT('',(2.55623464956316,-0.509888470297935,6.40001295625876));
#22890=CARTESIAN_POINT('',(2.93123464956316,-0.5099,6.4));
#22891=CARTESIAN_POINT('',(2.6,-0.132288496556896,5.90755938055567));
#22892=CARTESIAN_POINT('Ctrl Pts',(2.6,-0.132288496556895,5.90755938055567));
#22893=CARTESIAN_POINT('Ctrl Pts',(2.59602705447461,-0.214239653399634,
5.92957461427473));
#22894=CARTESIAN_POINT('Ctrl Pts',(2.58808116342382,-0.366850103542102,
6.0153123398751));
#22895=CARTESIAN_POINT('Ctrl Pts',(2.57766961356943,-0.488635125282487,
6.20977428615126));
#22896=CARTESIAN_POINT('Ctrl Pts',(2.57123100924044,-0.509836321405008,
6.34733983573258));
#22897=CARTESIAN_POINT('Ctrl Pts',(2.56876535043684,-0.509867809550215,
6.40001069114481));
#22898=CARTESIAN_POINT('',(2.6,0.132303594671782,5.90751949357016));
#22899=CARTESIAN_POINT('Origin',(2.6,0.,6.4));
#22900=CARTESIAN_POINT('Ctrl Pts',(2.6,0.132303594671782,5.90751949357016));
#22901=CARTESIAN_POINT('Ctrl Pts',(2.59622409987445,0.0544270437755129,
5.88663631098165));
#22902=CARTESIAN_POINT('Ctrl Pts',(2.58847525422351,-0.115765473878103,
5.88226868015152));
#22903=CARTESIAN_POINT('Ctrl Pts',(2.57675346304718,-0.347023432783479,
5.99732787846002));
#22904=CARTESIAN_POINT('Ctrl Pts',(2.56594091302711,-0.483490786405975,
6.19264042843836));
#22905=CARTESIAN_POINT('Ctrl Pts',(2.55910130853244,-0.509829655724409,
6.3387818547688));
#22906=CARTESIAN_POINT('Ctrl Pts',(2.55623464956316,-0.509888470297935,
6.40001295625876));
#22907=CARTESIAN_POINT('Origin',(2.,-0.574456264653803,6.8));
#22908=CARTESIAN_POINT('',(2.,0.574456264653803,6.8));
#22909=CARTESIAN_POINT('',(2.,0.360555127546398,7.));
#22910=CARTESIAN_POINT('Origin',(2.,0.,6.4));
#22911=CARTESIAN_POINT('',(2.,0.574456264653803,7.));
#22912=CARTESIAN_POINT('',(2.,0.574456264653803,6.8));
#22913=CARTESIAN_POINT('',(2.,0.,7.));
#22914=CARTESIAN_POINT('Origin',(-2.,0.574456264653803,6.8));
#22915=CARTESIAN_POINT('',(-2.,0.574456264653803,6.8));
#22916=CARTESIAN_POINT('',(-2.,0.360555127546398,7.));
#22917=CARTESIAN_POINT('Origin',(-2.,0.,6.4));
#22918=CARTESIAN_POINT('',(-2.,0.574456264653803,7.));
#22919=CARTESIAN_POINT('',(-2.,0.574456264653803,7.));
#22920=CARTESIAN_POINT('',(-2.,0.574456264653803,6.8));
#22921=CARTESIAN_POINT('Origin',(2.33023603954621,-0.574456264653802,6.8));
#22922=CARTESIAN_POINT('',(2.33023603954621,-0.574456264653803,6.8));
#22923=CARTESIAN_POINT('',(2.,-0.574456264653803,6.8));
#22924=CARTESIAN_POINT('',(2.,-0.574456264653803,6.8));
#22925=CARTESIAN_POINT('',(2.,-0.574456264653803,7.));
#22926=CARTESIAN_POINT('',(2.,-0.574456264653803,6.8));
#22927=CARTESIAN_POINT('',(2.33023603954621,-0.574456264653802,7.));
#22928=CARTESIAN_POINT('',(2.33023603954621,-0.574456264653802,7.));
#22929=CARTESIAN_POINT('',(2.33023603954621,-0.574456264653802,6.8));
#22930=CARTESIAN_POINT('Origin',(-2.,-0.574456264653803,6.8));
#22931=CARTESIAN_POINT('',(-2.,-0.574456264653803,6.8));
#22932=CARTESIAN_POINT('',(-2.33023603954621,-0.574456264653803,6.8));
#22933=CARTESIAN_POINT('',(-2.,-0.574456264653803,6.8));
#22934=CARTESIAN_POINT('',(-2.33023603954621,-0.574456264653803,7.));
#22935=CARTESIAN_POINT('',(-2.33023603954621,-0.574456264653803,6.8));
#22936=CARTESIAN_POINT('',(-2.,-0.574456264653803,7.));
#22937=CARTESIAN_POINT('',(-2.,-0.574456264653803,7.));
#22938=CARTESIAN_POINT('',(-2.,-0.574456264653803,6.8));
#22939=CARTESIAN_POINT('Origin',(-2.,0.574456264653803,6.8));
#22940=CARTESIAN_POINT('',(-2.,-0.360555127546398,7.));
#22941=CARTESIAN_POINT('Origin',(-2.,0.,6.4));
#22942=CARTESIAN_POINT('',(-2.,0.574456264653803,7.));
#22943=CARTESIAN_POINT('Origin',(-2.33023603954621,0.574456264653802,6.8));
#22944=CARTESIAN_POINT('',(-2.33023603954621,0.574456264653803,6.8));
#22945=CARTESIAN_POINT('',(-2.,0.574456264653803,6.8));
#22946=CARTESIAN_POINT('',(-2.33023603954621,0.574456264653802,7.));
#22947=CARTESIAN_POINT('',(-2.33023603954621,0.574456264653802,7.));
#22948=CARTESIAN_POINT('',(-2.33023603954621,0.574456264653802,6.8));
#22949=CARTESIAN_POINT('Origin',(2.,0.574456264653803,6.8));
#22950=CARTESIAN_POINT('',(2.33023603954621,0.574456264653803,6.8));
#22951=CARTESIAN_POINT('',(2.,0.574456264653803,6.8));
#22952=CARTESIAN_POINT('',(2.33023603954621,0.574456264653803,7.));
#22953=CARTESIAN_POINT('',(2.33023603954621,0.574456264653803,6.8));
#22954=CARTESIAN_POINT('',(2.,0.574456264653803,7.));
#22955=CARTESIAN_POINT('Origin',(2.,-0.574456264653803,6.8));
#22956=CARTESIAN_POINT('',(2.,-0.360555127546398,7.));
#22957=CARTESIAN_POINT('Origin',(2.,0.,6.4));
#22958=CARTESIAN_POINT('',(2.,0.,7.));
#22959=CARTESIAN_POINT('Origin',(0.,0.,7.));
#22960=CARTESIAN_POINT('',(2.,0.,7.));
#22961=CARTESIAN_POINT('Origin',(0.,0.,7.));
#22962=CARTESIAN_POINT('',(-2.,0.,7.));
#22963=CARTESIAN_POINT('Origin',(0.,0.,7.));
#22964=CARTESIAN_POINT('',(-0.6,7.34788079488412E-17,7.));
#22965=CARTESIAN_POINT('Origin',(0.,0.,7.));
#22966=CARTESIAN_POINT('Origin',(-2.,0.,6.4));
#22967=CARTESIAN_POINT('Origin',(-2.,0.,6.4));
#22968=CARTESIAN_POINT('Origin',(2.93123464956316,0.,6.4));
#22969=CARTESIAN_POINT('Ctrl Pts',(2.55623464956316,-0.509888470297935,
6.40001295625876));
#22970=CARTESIAN_POINT('Ctrl Pts',(2.55512836300704,-0.509911167721204,
6.42364295379955));
#22971=CARTESIAN_POINT('Ctrl Pts',(2.55004913092554,-0.502507177574701,
6.53211994282295));
#22972=CARTESIAN_POINT('Ctrl Pts',(2.54099695331864,-0.426919346618493,
6.7167170754366));
#22973=CARTESIAN_POINT('Ctrl Pts',(2.52907811674246,-0.223174193283009,
6.88245524211623));
#22974=CARTESIAN_POINT('Ctrl Pts',(2.51715928016628,0.0350524704178637,
6.93041600240246));
#22975=CARTESIAN_POINT('Ctrl Pts',(2.5052404435901,0.284722093726431,6.84889099741939));
#22976=CARTESIAN_POINT('Ctrl Pts',(2.49332160701392,0.464885050226796,6.6577822578485));
#22977=CARTESIAN_POINT('Ctrl Pts',(2.48140277043774,0.531559769507257,6.40374342750432));
#22978=CARTESIAN_POINT('Ctrl Pts',(2.46948393386156,0.468469545343797,6.14879075163119));
#22979=CARTESIAN_POINT('Ctrl Pts',(2.45756509728538,0.291016032073294,5.95516354586177));
#22980=CARTESIAN_POINT('Ctrl Pts',(2.4456462607092,0.0425193718295788,5.87013029471448));
#22981=CARTESIAN_POINT('Ctrl Pts',(2.43372742413302,-0.216357163144678,
5.91444940567057));
#22982=CARTESIAN_POINT('Ctrl Pts',(2.42180858755684,-0.422416354717456,
6.07730165027367));
#22983=CARTESIAN_POINT('Ctrl Pts',(2.41264432936689,-0.501564565860727,
6.26308799447805));
#22984=CARTESIAN_POINT('Ctrl Pts',(2.40745301670233,-0.50990474610345,6.37396275616984));
#22985=CARTESIAN_POINT('Ctrl Pts',(2.40623464956316,-0.509881639433629,
6.39998778127036));
#22986=CARTESIAN_POINT('Ctrl Pts',(2.56876535043684,-0.509867809550215,
6.40001069114481));
#22987=CARTESIAN_POINT('Ctrl Pts',(2.56725806371505,-0.509887058630054,
6.4322090151272));
#22988=CARTESIAN_POINT('Ctrl Pts',(2.56177783146786,-0.498968432159698,
6.54926324266892));
#22989=CARTESIAN_POINT('Ctrl Pts',(2.55232465369528,-0.410425773087965,
6.73782039475945));
#22990=CARTESIAN_POINT('Ctrl Pts',(2.54040581711911,-0.19858907062663,6.89308342832313));
#22991=CARTESIAN_POINT('Ctrl Pts',(2.52848698054292,0.0617246536500735,
6.92797742227401));
#22992=CARTESIAN_POINT('Ctrl Pts',(2.51656814396674,0.306971377021502,6.8339796336226));
#22993=CARTESIAN_POINT('Ctrl Pts',(2.50464930739056,0.477279320739804,6.63403891232169));
#22994=CARTESIAN_POINT('Ctrl Pts',(2.49273047081439,0.531073600862929,6.3769640630774));
#22995=CARTESIAN_POINT('Ctrl Pts',(2.48081163423821,0.455221493256117,6.12551290982166));
#22996=CARTESIAN_POINT('Ctrl Pts',(2.46889279766203,0.268240284898955,5.94106977614238));
#22997=CARTESIAN_POINT('Ctrl Pts',(2.45697396108585,0.0157759417689948,
5.86866121228054));
#22998=CARTESIAN_POINT('Ctrl Pts',(2.44505512450967,-0.240539628301038,
5.92596363104932));
#22999=CARTESIAN_POINT('Ctrl Pts',(2.43313628793349,-0.438134411540293,
6.09898832463164));
#23000=CARTESIAN_POINT('Ctrl Pts',(2.42437302990921,-0.504774712912163,
6.28023194354175));
#23001=CARTESIAN_POINT('Ctrl Pts',(2.41958271741033,-0.509925751376541,
6.3825301408573));
#23002=CARTESIAN_POINT('Ctrl Pts',(2.41876535043684,-0.509907683680876,
6.3999870064905));
#23003=CARTESIAN_POINT('Ctrl Pts',(2.6,0.322335278395778,6.67898325810255));
#23004=CARTESIAN_POINT('Ctrl Pts',(2.59602705447461,0.368763212726337,6.62534075195518));
#23005=CARTESIAN_POINT('Ctrl Pts',(2.58808116342382,0.434258099467944,6.4944682619995));
#23006=CARTESIAN_POINT('Ctrl Pts',(2.57616232684764,0.426482264300449,6.27500430516079));
#23007=CARTESIAN_POINT('Ctrl Pts',(2.56424349027146,0.314584469477882,6.08608472387891));
#23008=CARTESIAN_POINT('Ctrl Pts',(2.55232465369528,0.125891708691813,5.97378227942249));
#23009=CARTESIAN_POINT('Ctrl Pts',(2.5404058171191,-0.0935351747046863,
5.96553560214966));
#23010=CARTESIAN_POINT('Ctrl Pts',(2.52848698054292,-0.290127651295543,
6.06334746928321));
#23011=CARTESIAN_POINT('Ctrl Pts',(2.51656814396674,-0.415894108139653,
6.24334485866553));
#23012=CARTESIAN_POINT('Ctrl Pts',(2.50464930739057,-0.440131934448267,
6.46158434769009));
#23013=CARTESIAN_POINT('Ctrl Pts',(2.49273047081439,-0.356924333130935,
6.66479013386668));
#23014=CARTESIAN_POINT('Ctrl Pts',(2.48081163423821,-0.186583954886344,
6.80335491216739));
#23015=CARTESIAN_POINT('Ctrl Pts',(2.46889279766203,0.0293054876233287,
6.8434523275626));
#23016=CARTESIAN_POINT('Ctrl Pts',(2.45697396108585,0.238040848314528,6.77529365012726));
#23017=CARTESIAN_POINT('Ctrl Pts',(2.44505512450967,0.388665418536347,6.61551789864839));
#23018=CARTESIAN_POINT('Ctrl Pts',(2.43313628793349,0.444408569799851,6.40312967865285));
#23019=CARTESIAN_POINT('Ctrl Pts',(2.42121745135731,0.391662222357444,6.18997744149907));
#23020=CARTESIAN_POINT('Ctrl Pts',(2.40929861478113,0.243302872078535,6.0280961357146));
#23021=CARTESIAN_POINT('Ctrl Pts',(2.39737977820495,0.0355481627984888,
5.95700440211175));
#23022=CARTESIAN_POINT('Ctrl Pts',(2.38546094162877,-0.180884602174105,
5.99405723011839));
#23023=CARTESIAN_POINT('Ctrl Pts',(2.37354210505259,-0.353159623487059,
6.13020924399229));
#23024=CARTESIAN_POINT('Ctrl Pts',(2.36162326847641,-0.439220937561425,
6.33222286740014));
#23025=CARTESIAN_POINT('Ctrl Pts',(2.34970443190023,-0.418059163834771,
6.55078231736932));
#23026=CARTESIAN_POINT('Ctrl Pts',(2.33778559532405,-0.29484033726761,6.73253262578912));
#23027=CARTESIAN_POINT('Ctrl Pts',(2.32586675874787,-0.099644770368915,
6.83310471186003));
#23028=CARTESIAN_POINT('Ctrl Pts',(2.3139479221717,0.119876185075048,6.82794680971604));
#23029=CARTESIAN_POINT('Ctrl Pts',(2.30202908559551,0.310132837249173,6.71831807199288));
#23030=CARTESIAN_POINT('Ctrl Pts',(2.29011024901934,0.424679527547163,6.53098118406136));
#23031=CARTESIAN_POINT('Ctrl Pts',(2.27819141244315,0.435552994685514,6.31166902859576));
#23032=CARTESIAN_POINT('Ctrl Pts',(2.26627257586698,0.340098796199685,6.11392032482827));
#23033=CARTESIAN_POINT('Ctrl Pts',(2.2543537392908,0.16161931364965,5.98600969928979));
#23034=CARTESIAN_POINT('Ctrl Pts',(2.24243490271462,-0.0563148495252739,
5.95916283101918));
#23035=CARTESIAN_POINT('Ctrl Pts',(2.23051606613844,-0.260501371261513,
6.03993360741091));
#23036=CARTESIAN_POINT('Ctrl Pts',(2.21859722956226,-0.401094017530737,
6.20860417742001));
#23037=CARTESIAN_POINT('Ctrl Pts',(2.20667839298608,-0.44377116171621,6.42399850480546));
#23038=CARTESIAN_POINT('Ctrl Pts',(2.1947595564099,-0.378114410354912,6.63353428436548));
#23039=CARTESIAN_POINT('Ctrl Pts',(2.18284071983372,-0.220151966921295,
6.78605943828148));
#23040=CARTESIAN_POINT('Ctrl Pts',(2.17092188325754,-0.00844577862671016,
6.84433931427905));
#23041=CARTESIAN_POINT('Ctrl Pts',(2.15900304668136,0.205322181057602,6.79414666881739));
#23042=CARTESIAN_POINT('Ctrl Pts',(2.14708421010518,0.368966714730599,6.64773436383049));
#23043=CARTESIAN_POINT('Ctrl Pts',(2.135165373529,0.442538599255273,6.44084520364718));
#23044=CARTESIAN_POINT('Ctrl Pts',(2.12324653695282,0.408077698331108,6.22398416943617));
#23045=CARTESIAN_POINT('Ctrl Pts',(2.11132770037664,0.273995984823229,6.05009380941852));
#23046=CARTESIAN_POINT('Ctrl Pts',(2.09940886380046,0.0730271011145798,
5.96161967407919));
#23047=CARTESIAN_POINT('Ctrl Pts',(2.08749002722429,-0.145771140848075,
5.98017031606292));
#23048=CARTESIAN_POINT('Ctrl Pts',(2.07557119064811,-0.328978055262558,
6.10119490525287));
#23049=CARTESIAN_POINT('Ctrl Pts',(2.06365235407193,-0.431879950098104,
6.29519514237415));
#23050=CARTESIAN_POINT('Ctrl Pts',(2.05570646302114,-0.430162668703658,
6.44153119316515));
#23051=CARTESIAN_POINT('Ctrl Pts',(2.05173351749575,-0.411845039474987,
6.51006976632957));
#23052=CARTESIAN_POINT('Ctrl Pts',(2.61608882750142,0.34340590883904,6.69722002436839));
#23053=CARTESIAN_POINT('Ctrl Pts',(2.61211588197602,0.392868775775771,6.64007097860578));
#23054=CARTESIAN_POINT('Ctrl Pts',(2.60416999092524,0.462644976561947,6.5006435272299));
#23055=CARTESIAN_POINT('Ctrl Pts',(2.59225115434906,0.454360845343155,6.26683350205768));
#23056=CARTESIAN_POINT('Ctrl Pts',(2.58033231777288,0.335148439802654,6.065564497838));
#23057=CARTESIAN_POINT('Ctrl Pts',(2.5684134811967,0.134121083034322,5.94592099125275));
#23058=CARTESIAN_POINT('Ctrl Pts',(2.55649464462052,-0.0996494452538391,
5.9371352396035));
#23059=CARTESIAN_POINT('Ctrl Pts',(2.54457580804434,-0.309092911791522,
6.04134093900881));
#23060=CARTESIAN_POINT('Ctrl Pts',(2.53265697146816,-0.443080555430665,
6.23310451945562));
#23061=CARTESIAN_POINT('Ctrl Pts',(2.52073813489198,-0.468902776359187,
6.46561003497361));
#23062=CARTESIAN_POINT('Ctrl Pts',(2.5088192983158,-0.380256004293454,6.68209911438999));
#23063=CARTESIAN_POINT('Ctrl Pts',(2.49690046173962,-0.198780701018566,
6.829721688817));
#23064=CARTESIAN_POINT('Ctrl Pts',(2.48498162516344,0.0312211485548406,
6.87244021917589));
#23065=CARTESIAN_POINT('Ctrl Pts',(2.47306278858727,0.253601263451829,6.79982609922463));
#23066=CARTESIAN_POINT('Ctrl Pts',(2.46114395201108,0.414071962433164,6.62960601838176));
#23067=CARTESIAN_POINT('Ctrl Pts',(2.44922511543491,0.473458969702319,6.40333426160334));
#23068=CARTESIAN_POINT('Ctrl Pts',(2.43730627885873,0.417264663352895,6.17624854487645));
#23069=CARTESIAN_POINT('Ctrl Pts',(2.42538744228255,0.259207258743454,6.00378527243032));
#23070=CARTESIAN_POINT('Ctrl Pts',(2.41346860570637,0.0378718991421855,
5.92804636631267));
#23071=CARTESIAN_POINT('Ctrl Pts',(2.40154976913019,-0.192708789164296,
5.96752128863578));
#23072=CARTESIAN_POINT('Ctrl Pts',(2.38963093255401,-0.376245200563858,
6.11257337941941));
#23073=CARTESIAN_POINT('Ctrl Pts',(2.37771209597783,-0.467932228811824,
6.32779236596503));
#23074=CARTESIAN_POINT('Ctrl Pts',(2.36579325940165,-0.445387137950485,
6.56063875785105));
#23075=CARTESIAN_POINT('Ctrl Pts',(2.35387442282547,-0.314113659806958,
6.75426984333229));
#23076=CARTESIAN_POINT('Ctrl Pts',(2.34195558624929,-0.106158417098793,
6.86141619353295));
#23077=CARTESIAN_POINT('Ctrl Pts',(2.33003674967311,0.127712332602043,6.85592112615381));
#23078=CARTESIAN_POINT('Ctrl Pts',(2.31811791309693,0.330405810268198,6.73912610297154));
#23079=CARTESIAN_POINT('Ctrl Pts',(2.30619907652075,0.452440266074759,6.53954325067136));
#23080=CARTESIAN_POINT('Ctrl Pts',(2.29428023994457,0.464024517365714,6.30589494992706));
#23081=CARTESIAN_POINT('Ctrl Pts',(2.28236140336839,0.362330604286552,6.09521967517282));
#23082=CARTESIAN_POINT('Ctrl Pts',(2.27044256679221,0.172184154232268,5.95894770137019));
#23083=CARTESIAN_POINT('Ctrl Pts',(2.25852373021603,-0.0599960766894875,
5.93034588886046));
#23084=CARTESIAN_POINT('Ctrl Pts',(2.24660489363985,-0.277530001050755,
6.01639654398105));
#23085=CARTESIAN_POINT('Ctrl Pts',(2.23468605706368,-0.427313002490913,
6.19609288586657));
#23086=CARTESIAN_POINT('Ctrl Pts',(2.2227672204875,-0.472779895096048,6.42556725529552));
#23087=CARTESIAN_POINT('Ctrl Pts',(2.21084838391132,-0.402831248814268,
6.64880011138319));
#23088=CARTESIAN_POINT('Ctrl Pts',(2.19892954733514,-0.234543009563112,
6.81129563269882));
#23089=CARTESIAN_POINT('Ctrl Pts',(2.18701071075896,-0.00899786799506803,
6.8733851870398));
#23090=CARTESIAN_POINT('Ctrl Pts',(2.17509187418278,0.218743820229089,6.81991151478903));
#23091=CARTESIAN_POINT('Ctrl Pts',(2.1631730376066,0.393085580436657,6.66392843124485));
#23092=CARTESIAN_POINT('Ctrl Pts',(2.15125420103042,0.471466761658698,6.44351520053897));
#23093=CARTESIAN_POINT('Ctrl Pts',(2.13933536445424,0.43475319726025,6.2124782476009));
#23094=CARTESIAN_POINT('Ctrl Pts',(2.12741652787806,0.291906739636914,6.02722090494389));
#23095=CARTESIAN_POINT('Ctrl Pts',(2.11549769130188,0.0778007860416099,
5.93296333249894));
#23096=CARTESIAN_POINT('Ctrl Pts',(2.1035788547257,-0.155300007354369,5.95272660539192));
#23097=CARTESIAN_POINT('Ctrl Pts',(2.09166001814952,-0.350482915235934,
6.08166241176561));
#23098=CARTESIAN_POINT('Ctrl Pts',(2.07974118157334,-0.46011137071598,6.28834418757117));
#23099=CARTESIAN_POINT('Ctrl Pts',(2.07179529052256,-0.458281832910106,
6.44424603228361));
#23100=CARTESIAN_POINT('Ctrl Pts',(2.06782234499716,-0.438766804507522,
6.51726488124485));
#23101=CARTESIAN_POINT('Ctrl Pts',(2.63217765500284,0.364476539282301,6.71545679063422));
#23102=CARTESIAN_POINT('Ctrl Pts',(2.62820470947744,0.416974338825206,6.65480120525638));
#23103=CARTESIAN_POINT('Ctrl Pts',(2.62025881842666,0.49103185365595,6.5068187924603));
#23104=CARTESIAN_POINT('Ctrl Pts',(2.60833998185048,0.482239426385862,6.25866269895458));
#23105=CARTESIAN_POINT('Ctrl Pts',(2.5964211452743,0.355712410127426,6.04504427179708));
#23106=CARTESIAN_POINT('Ctrl Pts',(2.58450230869812,0.142350457376832,5.91805970308301));
#23107=CARTESIAN_POINT('Ctrl Pts',(2.57258347212194,-0.105763715802992,
5.90873487705734));
#23108=CARTESIAN_POINT('Ctrl Pts',(2.56066463554576,-0.3280581722875,6.01933440873442));
#23109=CARTESIAN_POINT('Ctrl Pts',(2.54874579896958,-0.470267002721677,
6.2228641802457));
#23110=CARTESIAN_POINT('Ctrl Pts',(2.5368269623934,-0.497673618270107,6.46963572225713));
#23111=CARTESIAN_POINT('Ctrl Pts',(2.52490812581722,-0.403587675455974,
6.69940809491329));
#23112=CARTESIAN_POINT('Ctrl Pts',(2.51298928924104,-0.210977447150787,
6.85608846546662));
#23113=CARTESIAN_POINT('Ctrl Pts',(2.50107045266486,0.0331368094863519,
6.90142811078917));
#23114=CARTESIAN_POINT('Ctrl Pts',(2.48915161608868,0.26916167858913,6.82435854832202));
#23115=CARTESIAN_POINT('Ctrl Pts',(2.4772327795125,0.43947850632998,6.64369413811513));
#23116=CARTESIAN_POINT('Ctrl Pts',(2.46531394293632,0.502509369604788,6.40353884455383));
#23117=CARTESIAN_POINT('Ctrl Pts',(2.45339510636014,0.442867104348346,6.16251964825382));
#23118=CARTESIAN_POINT('Ctrl Pts',(2.44147626978397,0.275111645408374,5.97947440914605));
#23119=CARTESIAN_POINT('Ctrl Pts',(2.42955743320778,0.0401956354858822,
5.89908833051357));
#23120=CARTESIAN_POINT('Ctrl Pts',(2.41763859663161,-0.204532976154487,
5.94098534715318));
#23121=CARTESIAN_POINT('Ctrl Pts',(2.40571976005543,-0.399330777640657,
6.09493751484654));
#23122=CARTESIAN_POINT('Ctrl Pts',(2.39380092347925,-0.496643520062223,
6.32336186452993));
#23123=CARTESIAN_POINT('Ctrl Pts',(2.38188208690307,-0.472715112066199,
6.57049519833277));
#23124=CARTESIAN_POINT('Ctrl Pts',(2.36996325032689,-0.333386982346306,
6.77600706087547));
#23125=CARTESIAN_POINT('Ctrl Pts',(2.35804441375071,-0.112672063828671,
6.88972767520587));
#23126=CARTESIAN_POINT('Ctrl Pts',(2.34612557717453,0.135548480129038,6.88389544259157));
#23127=CARTESIAN_POINT('Ctrl Pts',(2.33420674059835,0.350678783287223,6.7599341339502));
#23128=CARTESIAN_POINT('Ctrl Pts',(2.32228790402217,0.480201004602356,6.54810531728136));
#23129=CARTESIAN_POINT('Ctrl Pts',(2.31036906744599,0.492496040045916,6.30012087125837));
#23130=CARTESIAN_POINT('Ctrl Pts',(2.29845023086981,0.384562412373419,6.07651902551736));
#23131=CARTESIAN_POINT('Ctrl Pts',(2.28653139429363,0.182748994814887,5.9318857034506));
#23132=CARTESIAN_POINT('Ctrl Pts',(2.27461255771745,-0.0636773038537012,
5.90152894670173));
#23133=CARTESIAN_POINT('Ctrl Pts',(2.26269372114127,-0.294558630839998,
5.99285948055119));
#23134=CARTESIAN_POINT('Ctrl Pts',(2.25077488456509,-0.453531987451089,
6.18358159431314));
#23135=CARTESIAN_POINT('Ctrl Pts',(2.23885604798891,-0.501788628475886,
6.42713600578558));
#23136=CARTESIAN_POINT('Ctrl Pts',(2.22693721141274,-0.427548087273624,
6.6640659384009));
#23137=CARTESIAN_POINT('Ctrl Pts',(2.21501837483655,-0.24893405220493,6.83653182711616));
#23138=CARTESIAN_POINT('Ctrl Pts',(2.20309953826038,-0.00954995736342605,
6.90243105980056));
#23139=CARTESIAN_POINT('Ctrl Pts',(2.1911807016842,0.232165459400577,6.84567636076067));
#23140=CARTESIAN_POINT('Ctrl Pts',(2.17926186510802,0.417204446142715,6.68012249865921));
#23141=CARTESIAN_POINT('Ctrl Pts',(2.16734302853184,0.500394924062124,6.44618519743075));
#23142=CARTESIAN_POINT('Ctrl Pts',(2.15542419195566,0.461428696189393,6.20097232576562));
#23143=CARTESIAN_POINT('Ctrl Pts',(2.14350535537948,0.309817494450599,6.00434800046925));
#23144=CARTESIAN_POINT('Ctrl Pts',(2.1315865188033,0.0825744709686401,5.90430699091869));
#23145=CARTESIAN_POINT('Ctrl Pts',(2.11966768222712,-0.164828873860662,
5.92528289472092));
#23146=CARTESIAN_POINT('Ctrl Pts',(2.10774884565094,-0.371987775209309,
6.06212991827835));
#23147=CARTESIAN_POINT('Ctrl Pts',(2.09583000907476,-0.488342791333856,
6.2814932327682));
#23148=CARTESIAN_POINT('Ctrl Pts',(2.08788411802398,-0.486400997116553,
6.44696087140208));
#23149=CARTESIAN_POINT('Ctrl Pts',(2.08391117249858,-0.465688569540057,
6.52445999616013));
#23150=CARTESIAN_POINT('Ctrl Pts',(2.64826648250425,0.385547169725563,6.73369355690005));
#23151=CARTESIAN_POINT('Ctrl Pts',(2.64429353697886,0.44107990187464,6.66953143190698));
#23152=CARTESIAN_POINT('Ctrl Pts',(2.63634764592807,0.519418730749953,6.5129940576907));
#23153=CARTESIAN_POINT('Ctrl Pts',(2.62442880935189,0.510118007428568,6.25049189585148));
#23154=CARTESIAN_POINT('Ctrl Pts',(2.61250997277571,0.376276380452198,6.02452404575617));
#23155=CARTESIAN_POINT('Ctrl Pts',(2.60059113619954,0.150579831719341,5.89019841491327));
#23156=CARTESIAN_POINT('Ctrl Pts',(2.58867229962336,-0.111877986352145,
5.88033451451117));
#23157=CARTESIAN_POINT('Ctrl Pts',(2.57675346304718,-0.347023432783479,
5.99732787846002));
#23158=CARTESIAN_POINT('Ctrl Pts',(2.564834626471,-0.497453450012689,6.21262384103579));
#23159=CARTESIAN_POINT('Ctrl Pts',(2.55291578989482,-0.526444460181026,
6.47366140954065));
#23160=CARTESIAN_POINT('Ctrl Pts',(2.54099695331864,-0.426919346618493,
6.7167170754366));
#23161=CARTESIAN_POINT('Ctrl Pts',(2.52907811674246,-0.223174193283009,
6.88245524211623));
#23162=CARTESIAN_POINT('Ctrl Pts',(2.51715928016628,0.0350524704178637,
6.93041600240246));
#23163=CARTESIAN_POINT('Ctrl Pts',(2.5052404435901,0.284722093726431,6.84889099741939));
#23164=CARTESIAN_POINT('Ctrl Pts',(2.49332160701392,0.464885050226796,6.6577822578485));
#23165=CARTESIAN_POINT('Ctrl Pts',(2.48140277043774,0.531559769507257,6.40374342750432));
#23166=CARTESIAN_POINT('Ctrl Pts',(2.46948393386156,0.468469545343797,6.14879075163119));
#23167=CARTESIAN_POINT('Ctrl Pts',(2.45756509728538,0.291016032073294,5.95516354586177));
#23168=CARTESIAN_POINT('Ctrl Pts',(2.4456462607092,0.0425193718295788,5.87013029471448));
#23169=CARTESIAN_POINT('Ctrl Pts',(2.43372742413302,-0.216357163144678,
5.91444940567057));
#23170=CARTESIAN_POINT('Ctrl Pts',(2.42180858755684,-0.422416354717456,
6.07730165027367));
#23171=CARTESIAN_POINT('Ctrl Pts',(2.40988975098066,-0.525354811312622,
6.31893136309484));
#23172=CARTESIAN_POINT('Ctrl Pts',(2.39797091440449,-0.500043086181913,
6.58035163881449));
#23173=CARTESIAN_POINT('Ctrl Pts',(2.38605207782831,-0.352660304885654,
6.79774427841866));
#23174=CARTESIAN_POINT('Ctrl Pts',(2.37413324125213,-0.11918571055855,6.91803915687878));
#23175=CARTESIAN_POINT('Ctrl Pts',(2.36221440467595,0.143384627656033,6.91186975902934));
#23176=CARTESIAN_POINT('Ctrl Pts',(2.35029556809977,0.370951756306248,6.78074216492885));
#23177=CARTESIAN_POINT('Ctrl Pts',(2.33837673152359,0.507961743129952,6.55666738389136));
#23178=CARTESIAN_POINT('Ctrl Pts',(2.32645789494741,0.520967562726117,6.29434679258967));
#23179=CARTESIAN_POINT('Ctrl Pts',(2.31453905837123,0.406794220460285,6.05781837586191));
#23180=CARTESIAN_POINT('Ctrl Pts',(2.30262022179505,0.193313835397505,5.904823705531));
#23181=CARTESIAN_POINT('Ctrl Pts',(2.29070138521887,-0.067358531017915,
5.872712004543));
#23182=CARTESIAN_POINT('Ctrl Pts',(2.27878254864269,-0.311587260629241,
5.96932241712133));
#23183=CARTESIAN_POINT('Ctrl Pts',(2.26686371206651,-0.479750972411266,
6.17107030275971));
#23184=CARTESIAN_POINT('Ctrl Pts',(2.25494487549033,-0.530797361855725,
6.42870475627563));
#23185=CARTESIAN_POINT('Ctrl Pts',(2.24302603891415,-0.45226492573298,6.67933176541862));
#23186=CARTESIAN_POINT('Ctrl Pts',(2.23110720233797,-0.263325094846747,
6.86176802153349));
#23187=CARTESIAN_POINT('Ctrl Pts',(2.2191883657618,-0.0101020467317839,
6.93147693256131));
#23188=CARTESIAN_POINT('Ctrl Pts',(2.20726952918561,0.245587098572064,6.87144120673232));
#23189=CARTESIAN_POINT('Ctrl Pts',(2.19535069260943,0.441323311848774,6.69631656607358));
#23190=CARTESIAN_POINT('Ctrl Pts',(2.18343185603326,0.529323086465549,6.44885519432254));
#23191=CARTESIAN_POINT('Ctrl Pts',(2.17151301945708,0.488104195118536,6.18946640393034));
#23192=CARTESIAN_POINT('Ctrl Pts',(2.1595941828809,0.327728249264285,5.98147509599461));
#23193=CARTESIAN_POINT('Ctrl Pts',(2.14767534630472,0.0873481558956701,
5.87565064933844));
#23194=CARTESIAN_POINT('Ctrl Pts',(2.13575650972854,-0.174357740366956,
5.89783918404992));
#23195=CARTESIAN_POINT('Ctrl Pts',(2.12383767315236,-0.393492635182685,
6.04259742479108));
#23196=CARTESIAN_POINT('Ctrl Pts',(2.11191883657618,-0.516574211951732,
6.27464227796523));
#23197=CARTESIAN_POINT('Ctrl Pts',(2.10397294552539,-0.514520161323001,
6.44967571052055));
#23198=CARTESIAN_POINT('Ctrl Pts',(2.1,-0.492610334572592,6.53165511107541));
#23199=CARTESIAN_POINT('Ctrl Pts',(2.1,-0.492610334572592,6.53165511107541));
#23200=CARTESIAN_POINT('Ctrl Pts',(2.1,-0.49635409029725,6.51110955003273));
#23201=CARTESIAN_POINT('Ctrl Pts',(2.1,-0.498800810154946,6.4903688790591));
#23202=CARTESIAN_POINT('Ctrl Pts',(2.1,-0.499959864786037,6.46955396620066));
#23203=CARTESIAN_POINT('Ctrl Pts',(2.1,-0.500651891757826,6.45712618175713));
#23204=CARTESIAN_POINT('Ctrl Pts',(2.1,-0.500884496511186,6.4446719156573));
#23205=CARTESIAN_POINT('Ctrl Pts',(2.1,-0.500656300483376,6.43221745273261));
#23206=CARTESIAN_POINT('Ctrl Pts',(2.1,-0.50051140625946,6.42430942840331));
#23207=CARTESIAN_POINT('Ctrl Pts',(2.1,-0.500180531457043,6.41639915136081));
#23208=CARTESIAN_POINT('Ctrl Pts',(2.1,-0.499663295188048,6.40850057461429));
#23209=CARTESIAN_POINT('Ctrl Pts',(2.1,-0.498282684765909,6.38741764205526));
#23210=CARTESIAN_POINT('Ctrl Pts',(2.1,-0.495579671230594,6.36646338372735));
#23211=CARTESIAN_POINT('Ctrl Pts',(2.1,-0.491553183641479,6.34576661740274));
#23212=CARTESIAN_POINT('Ctrl Pts',(2.1,-0.489189370076283,6.33361625162834));
#23213=CARTESIAN_POINT('Ctrl Pts',(2.1,-0.486369014762183,6.32155472699449));
#23214=CARTESIAN_POINT('Ctrl Pts',(2.1,-0.483088515935984,6.30960963623735));
#23215=CARTESIAN_POINT('Ctrl Pts',(2.1,-0.481387749157045,6.30341673247256));
#23216=CARTESIAN_POINT('Ctrl Pts',(2.1,-0.479562349371169,6.29725234131795));
#23217=CARTESIAN_POINT('Ctrl Pts',(2.1,-0.477614701955683,6.29113018362027));
#23218=CARTESIAN_POINT('Ctrl Pts',(2.1,-0.47691994455268,6.28894631073394));
#23219=CARTESIAN_POINT('Ctrl Pts',(2.1,-0.476209763711948,6.28676817605457));
#23220=CARTESIAN_POINT('Ctrl Pts',(2.1,-0.475484170198335,6.28459593876059));
#23221=CARTESIAN_POINT('Ctrl Pts',(2.1,-0.467396057947338,6.26038224508792));
#23222=CARTESIAN_POINT('Ctrl Pts',(2.1,-0.457396800695749,6.23689933548638));
#23223=CARTESIAN_POINT('Ctrl Pts',(2.1,-0.445625784567883,6.21434556134776));
#23224=CARTESIAN_POINT('Ctrl Pts',(2.1,-0.433955482728322,6.19198476012551));
#23225=CARTESIAN_POINT('Ctrl Pts',(2.1,-0.420542677238036,6.17053620507075));
#23226=CARTESIAN_POINT('Ctrl Pts',(2.1,-0.405485055004202,6.15022640072986));
#23227=CARTESIAN_POINT('Ctrl Pts',(2.1,-0.401547018955012,6.14491475587622));
#23228=CARTESIAN_POINT('Ctrl Pts',(2.1,-0.397496316871279,6.13968122438761));
#23229=CARTESIAN_POINT('Ctrl Pts',(2.1,-0.393334380355557,6.13453037462292));
#23230=CARTESIAN_POINT('Ctrl Pts',(2.1,-0.390073732726515,6.1304949680257));
#23231=CARTESIAN_POINT('Ctrl Pts',(2.1,-0.386745496616124,6.12651133724348));
#23232=CARTESIAN_POINT('Ctrl Pts',(2.1,-0.383357029508834,6.12258887921439));
#23233=CARTESIAN_POINT('Ctrl Pts',(2.1,-0.371904123413349,6.109331101568));
#23234=CARTESIAN_POINT('Ctrl Pts',(2.1,-0.35974458511925,6.09674730862358));
#23235=CARTESIAN_POINT('Ctrl Pts',(2.1,-0.346917810301558,6.08490712758635));
#23236=CARTESIAN_POINT('Ctrl Pts',(2.1,-0.328748103732818,6.06813497572237));
#23237=CARTESIAN_POINT('Ctrl Pts',(2.1,-0.309239814555027,6.0528527033034));
#23238=CARTESIAN_POINT('Ctrl Pts',(2.1,-0.288595198791424,6.03919240881688));
#23239=CARTESIAN_POINT('Ctrl Pts',(2.1,-0.278215530931981,6.03232430716481));
#23240=CARTESIAN_POINT('Ctrl Pts',(2.1,-0.26754829677856,6.02586696377693));
#23241=CARTESIAN_POINT('Ctrl Pts',(2.1,-0.256618135875702,6.01984205852923));
#23242=CARTESIAN_POINT('Ctrl Pts',(2.1,-0.251611498381037,6.01708230807514));
#23243=CARTESIAN_POINT('Ctrl Pts',(2.1,-0.246550009240434,6.01441370455151));
#23244=CARTESIAN_POINT('Ctrl Pts',(2.1,-0.241448312426713,6.01184414666615));
#23245=CARTESIAN_POINT('Ctrl Pts',(2.1,-0.219923137629529,6.00100261988527));
#23246=CARTESIAN_POINT('Ctrl Pts',(2.1,-0.197628752691819,5.99188954333672));
#23247=CARTESIAN_POINT('Ctrl Pts',(2.1,-0.174757433630984,5.98462368929255));
#23248=CARTESIAN_POINT('Ctrl Pts',(2.1,-0.165576347867032,5.98170700447212));
#23249=CARTESIAN_POINT('Ctrl Pts',(2.1,-0.156302149790289,5.97908854410605));
#23250=CARTESIAN_POINT('Ctrl Pts',(2.1,-0.146946980180942,5.97677835925102));
#23251=CARTESIAN_POINT('Ctrl Pts',(2.1,-0.136233092918806,5.97413264985985));
#23252=CARTESIAN_POINT('Ctrl Pts',(2.1,-0.125412970644963,5.971891235028));
#23253=CARTESIAN_POINT('Ctrl Pts',(2.1,-0.11450999527259,5.97005741415271));
#23254=CARTESIAN_POINT('Ctrl Pts',(2.1,-0.107187489851071,5.96882580875667));
#23255=CARTESIAN_POINT('Ctrl Pts',(2.1,-0.0998276196797078,5.96777809712117));
#23256=CARTESIAN_POINT('Ctrl Pts',(2.1,-0.0924376450671474,5.96691584094867));
#23257=CARTESIAN_POINT('Ctrl Pts',(2.1,-0.0866290251654119,5.96623809594594));
#23258=CARTESIAN_POINT('Ctrl Pts',(2.1,-0.0808012215405976,5.96567507726491));
#23259=CARTESIAN_POINT('Ctrl Pts',(2.1,-0.0749735051801638,5.96522838192892));
#23260=CARTESIAN_POINT('Ctrl Pts',(2.1,-0.0505591545770249,5.96335701828132));
#23261=CARTESIAN_POINT('Ctrl Pts',(2.1,-0.0260794227869884,5.96351369057634));
#23262=CARTESIAN_POINT('Ctrl Pts',(2.1,-0.00179128476957419,5.96570484843602));
#23263=CARTESIAN_POINT('Ctrl Pts',(2.1,0.0210365858903797,5.96776426806632));
#23264=CARTESIAN_POINT('Ctrl Pts',(2.1,0.0436964113942735,5.97162157501662));
#23265=CARTESIAN_POINT('Ctrl Pts',(2.1,0.065956881641688,5.97732901798388));
#23266=CARTESIAN_POINT('Ctrl Pts',(2.1,0.0673808531784219,5.97769411522767));
#23267=CARTESIAN_POINT('Ctrl Pts',(2.1,0.0688031806876158,5.97806679811498));
#23268=CARTESIAN_POINT('Ctrl Pts',(2.1,0.0702237992588386,5.97844708639908));
#23269=CARTESIAN_POINT('Ctrl Pts',(2.1,0.0736400801676868,5.97936159760649));
#23270=CARTESIAN_POINT('Ctrl Pts',(2.1,0.0770464797446285,5.9803200895664));
#23271=CARTESIAN_POINT('Ctrl Pts',(2.1,0.0804421690761142,5.98132232055468));
#23272=CARTESIAN_POINT('Ctrl Pts',(2.6,0.322335278395778,6.67898325810255));
#23273=CARTESIAN_POINT('Ctrl Pts',(2.6,0.339120601259259,6.66300806279478));
#23274=CARTESIAN_POINT('Ctrl Pts',(2.6,0.354506984127668,6.64569922647684));
#23275=CARTESIAN_POINT('Ctrl Pts',(2.6,0.368421126683117,6.62729272970921));
#23276=CARTESIAN_POINT('Ctrl Pts',(2.6,0.38257126416386,6.60857404411556));
#23277=CARTESIAN_POINT('Ctrl Pts',(2.6,0.395199756274692,6.58871918836577));
#23278=CARTESIAN_POINT('Ctrl Pts',(2.6,0.406199318727697,6.56793181289168));
#23279=CARTESIAN_POINT('Ctrl Pts',(2.6,0.409616043928294,6.56147476062801));
#23280=CARTESIAN_POINT('Ctrl Pts',(2.6,0.412875324168305,6.55492747138162));
#23281=CARTESIAN_POINT('Ctrl Pts',(2.6,0.415973133660165,6.54829542707107));
#23282=CARTESIAN_POINT('Ctrl Pts',(2.6,0.418485108810516,6.54291758490618));
#23283=CARTESIAN_POINT('Ctrl Pts',(2.6,0.420891069789125,6.53748311927057));
#23284=CARTESIAN_POINT('Ctrl Pts',(2.6,0.423182724471203,6.53201048034897));
#23285=CARTESIAN_POINT('Ctrl Pts',(2.6,0.42826857782987,6.51986509070635));
#23286=CARTESIAN_POINT('Ctrl Pts',(2.6,0.432799982024353,6.50751484134792));
#23287=CARTESIAN_POINT('Ctrl Pts',(2.6,0.436762141475896,6.49499689828687));
#23288=CARTESIAN_POINT('Ctrl Pts',(2.6,0.444013330815057,6.47208768012373));
#23289=CARTESIAN_POINT('Ctrl Pts',(2.6,0.449360985234842,6.44861814961569));
#23290=CARTESIAN_POINT('Ctrl Pts',(2.6,0.452831510630463,6.42482689824574));
#23291=CARTESIAN_POINT('Ctrl Pts',(2.6,0.45503518273379,6.40972021814094));
#23292=CARTESIAN_POINT('Ctrl Pts',(2.6,0.456481100414613,6.39448317547527));
#23293=CARTESIAN_POINT('Ctrl Pts',(2.6,0.457165780866727,6.37917321940029));
#23294=CARTESIAN_POINT('Ctrl Pts',(2.6,0.457426442969031,6.37334462399588));
#23295=CARTESIAN_POINT('Ctrl Pts',(2.6,0.457576507352781,6.36750526353339));
#23296=CARTESIAN_POINT('Ctrl Pts',(2.6,0.457615909648183,6.36167325953747));
#23297=CARTESIAN_POINT('Ctrl Pts',(2.6,0.457783624314556,6.33684951273631));
#23298=CARTESIAN_POINT('Ctrl Pts',(2.6,0.455954126792007,6.3120946330561));
#23299=CARTESIAN_POINT('Ctrl Pts',(2.6,0.452154218947823,6.28765697027383));
#23300=CARTESIAN_POINT('Ctrl Pts',(2.6,0.45115674289519,6.28124208222728));
#23301=CARTESIAN_POINT('Ctrl Pts',(2.6,0.450023226879442,6.27484896612481));
#23302=CARTESIAN_POINT('Ctrl Pts',(2.6,0.448753579228988,6.26848198366457));
#23303=CARTESIAN_POINT('Ctrl Pts',(2.6,0.444848441945282,6.24889864447494));
#23304=CARTESIAN_POINT('Ctrl Pts',(2.6,0.43965712635916,6.22956230418047));
#23305=CARTESIAN_POINT('Ctrl Pts',(2.6,0.433239797159997,6.21057739588651));
#23306=CARTESIAN_POINT('Ctrl Pts',(2.6,0.431489703713964,6.20539995172748));
#23307=CARTESIAN_POINT('Ctrl Pts',(2.6,0.429647959283524,6.200247760375));
#23308=CARTESIAN_POINT('Ctrl Pts',(2.6,0.427716565518185,6.19512580861043));
#23309=CARTESIAN_POINT('Ctrl Pts',(2.6,0.418824441384019,6.17154437652905));
#23310=CARTESIAN_POINT('Ctrl Pts',(2.6,0.408091715271334,6.14874908227563));
#23311=CARTESIAN_POINT('Ctrl Pts',(2.6,0.395672419048227,6.12693682894624));
#23312=CARTESIAN_POINT('Ctrl Pts',(2.6,0.383092367331082,6.10484223759245));
#23313=CARTESIAN_POINT('Ctrl Pts',(2.6,0.368781416403301,6.08375495651898));
#23314=CARTESIAN_POINT('Ctrl Pts',(2.6,0.352848584276632,6.06389024080292));
#23315=CARTESIAN_POINT('Ctrl Pts',(2.6,0.350477674538742,6.06093424104361));
#23316=CARTESIAN_POINT('Ctrl Pts',(2.6,0.348070766049518,6.05800535381594));
#23317=CARTESIAN_POINT('Ctrl Pts',(2.6,0.345628131270321,6.05510433731261));
#23318=CARTESIAN_POINT('Ctrl Pts',(2.6,0.341175445450433,6.04981606615654));
#23319=CARTESIAN_POINT('Ctrl Pts',(2.6,0.336604054215743,6.04462039757467));
#23320=CARTESIAN_POINT('Ctrl Pts',(2.6,0.331917615661801,6.03951989728949));
#23321=CARTESIAN_POINT('Ctrl Pts',(2.6,0.327197865992937,6.03438314274658));
#23322=CARTESIAN_POINT('Ctrl Pts',(2.6,0.322366287452079,6.02934835553984));
#23323=CARTESIAN_POINT('Ctrl Pts',(2.6,0.317432494385971,6.02442266645077));
#23324=CARTESIAN_POINT('Ctrl Pts',(2.6,0.305161639297739,6.01217196679398));
#23325=CARTESIAN_POINT('Ctrl Pts',(2.6,0.292249931632248,6.00058562939064));
#23326=CARTESIAN_POINT('Ctrl Pts',(2.6,0.278765100808516,5.98969663827542));
#23327=CARTESIAN_POINT('Ctrl Pts',(2.6,0.268765025516792,5.98162158472625));
#23328=CARTESIAN_POINT('Ctrl Pts',(2.6,0.258449546075054,5.97393011620472));
#23329=CARTESIAN_POINT('Ctrl Pts',(2.6,0.247843342520938,5.96663792616377));
#23330=CARTESIAN_POINT('Ctrl Pts',(2.6,0.241099106168833,5.96200099336216));
#23331=CARTESIAN_POINT('Ctrl Pts',(2.6,0.234236247932732,5.9575251822992));
#23332=CARTESIAN_POINT('Ctrl Pts',(2.6,0.227275760973999,5.95322352477529));
#23333=CARTESIAN_POINT('Ctrl Pts',(2.6,0.204751973270828,5.93930357615464));
#23334=CARTESIAN_POINT('Ctrl Pts',(2.6,0.181175137781382,5.92718033261133));
#23335=CARTESIAN_POINT('Ctrl Pts',(2.6,0.156760783265524,5.91698457674055));
#23336=CARTESIAN_POINT('Ctrl Pts',(2.6,0.152585729857118,5.91524101947092));
#23337=CARTESIAN_POINT('Ctrl Pts',(2.6,0.148386104006604,5.91355392287942));
#23338=CARTESIAN_POINT('Ctrl Pts',(2.6,0.144162892324896,5.91192406382743));
#23339=CARTESIAN_POINT('Ctrl Pts',(2.6,0.140229927621667,5.91040621944599));
#23340=CARTESIAN_POINT('Ctrl Pts',(2.6,0.136276507298105,5.90893801577657));
#23341=CARTESIAN_POINT('Ctrl Pts',(2.6,0.132303594671778,5.90751949357016));
#23342=CARTESIAN_POINT('Ctrl Pts',(2.3579681670589,-0.426284649716722,6.39998978457651));
#23343=CARTESIAN_POINT('Ctrl Pts',(2.35918653419807,-0.426303967962151,
6.37823165906101));
#23344=CARTESIAN_POINT('Ctrl Pts',(2.36040490133724,-0.424667502862756,
6.35647641245579));
#23345=CARTESIAN_POINT('Ctrl Pts',(2.36162326847641,-0.421350422927922,
6.33498050516036));
#23346=CARTESIAN_POINT('Ctrl Pts',(2.3655962140018,-0.41053383286997,6.26488499293085));
#23347=CARTESIAN_POINT('Ctrl Pts',(2.3695691595272,-0.381846728178515,6.19754711846157));
#23348=CARTESIAN_POINT('Ctrl Pts',(2.37354210505259,-0.338790672280628,
6.14118617891461));
#23349=CARTESIAN_POINT('Ctrl Pts',(2.37751505057798,-0.295734616382741,
6.08482523936765));
#23350=CARTESIAN_POINT('Ctrl Pts',(2.38148799610338,-0.238309609278423,
6.03944123474302));
#23351=CARTESIAN_POINT('Ctrl Pts',(2.38546094162877,-0.173524978230831,
6.01057376109627));
#23352=CARTESIAN_POINT('Ctrl Pts',(2.38943388715416,-0.10874034718324,5.98170628744951));
#23353=CARTESIAN_POINT('Ctrl Pts',(2.39340683267956,-0.036596092192376,
5.96935534478063));
#23354=CARTESIAN_POINT('Ctrl Pts',(2.39737977820495,0.0341018201830637,
5.97502849571334));
#23355=CARTESIAN_POINT('Ctrl Pts',(2.40135272373034,0.104799732558504,5.98070164664604));
#23356=CARTESIAN_POINT('Ctrl Pts',(2.40532566925574,0.174051302318518,6.00439889118032));
#23357=CARTESIAN_POINT('Ctrl Pts',(2.40929861478113,0.233403645578344,6.0432277310782));
#23358=CARTESIAN_POINT('Ctrl Pts',(2.41327156030652,0.29275598883817,6.08205657097609));
#23359=CARTESIAN_POINT('Ctrl Pts',(2.41724450583192,0.342209105597808,6.13601700623758));
#23360=CARTESIAN_POINT('Ctrl Pts',(2.42121745135731,0.375726721884694,6.19852259672729));
#23361=CARTESIAN_POINT('Ctrl Pts',(2.4251903968827,0.40924433817158,6.261028187217));
#23362=CARTESIAN_POINT('Ctrl Pts',(2.4291633424081,0.426826453985716,6.33207893293493));
#23363=CARTESIAN_POINT('Ctrl Pts',(2.43313628793349,0.426326986682199,6.40300234245982));
#23364=CARTESIAN_POINT('Ctrl Pts',(2.43710923345888,0.425827519378683,6.4739257519847));
#23365=CARTESIAN_POINT('Ctrl Pts',(2.44108217898427,0.407246468957515,6.54472182531654));
#23366=CARTESIAN_POINT('Ctrl Pts',(2.44505512450967,0.372851848709961,6.60674915389561));
#23367=CARTESIAN_POINT('Ctrl Pts',(2.44902807003506,0.338457228462407,6.66877648247468));
#23368=CARTESIAN_POINT('Ctrl Pts',(2.45300101556045,0.288249038388467,6.72203506630097));
#23369=CARTESIAN_POINT('Ctrl Pts',(2.45697396108585,0.228355716569631,6.76002413778667));
#23370=CARTESIAN_POINT('Ctrl Pts',(2.46094690661124,0.168462394750795,6.79801320927237));
#23371=CARTESIAN_POINT('Ctrl Pts',(2.46491985213663,0.0988839411870617,
6.82073276841748));
#23372=CARTESIAN_POINT('Ctrl Pts',(2.46889279766203,0.0281131406535831,
6.82540964542417));
#23373=CARTESIAN_POINT('Ctrl Pts',(2.47286574318742,-0.0426576598798955,
6.83008652243086));
#23374=CARTESIAN_POINT('Ctrl Pts',(2.47683868871281,-0.11462080738312,6.81672071729912));
#23375=CARTESIAN_POINT('Ctrl Pts',(2.48081163423821,-0.178992444175497,
6.78694368501647));
#23376=CARTESIAN_POINT('Ctrl Pts',(2.4847845797636,-0.243364080967874,6.75716665273382));
#23377=CARTESIAN_POINT('Ctrl Pts',(2.48875752528899,-0.300144207049405,
6.71097839330025));
#23378=CARTESIAN_POINT('Ctrl Pts',(2.49273047081439,-0.342402203643058,
6.65401663255403));
#23379=CARTESIAN_POINT('Ctrl Pts',(2.49670341633978,-0.384660200236712,
6.59705487180782));
#23380=CARTESIAN_POINT('Ctrl Pts',(2.50067636186517,-0.41239606734249,6.52931960974896));
#23381=CARTESIAN_POINT('Ctrl Pts',(2.50464930739057,-0.422224363177276,
6.45907873054876));
#23382=CARTESIAN_POINT('Ctrl Pts',(2.50575559394668,-0.424961101318294,
6.4395198063571));
#23383=CARTESIAN_POINT('Ctrl Pts',(2.50686188050279,-0.426309336731809,
6.41976660365709));
#23384=CARTESIAN_POINT('Ctrl Pts',(2.50796816705891,-0.426290360635438,
6.40001083203199));
#23385=CARTESIAN_POINT('Ctrl Pts',(2.6,-0.132288496556895,5.90755938055567));
#23386=CARTESIAN_POINT('Ctrl Pts',(2.59602705447461,-0.214239653399634,
5.92957461427473));
#23387=CARTESIAN_POINT('Ctrl Pts',(2.58808116342382,-0.366850103542102,
6.0153123398751));
#23388=CARTESIAN_POINT('Ctrl Pts',(2.57616232684764,-0.506266020658281,
6.23792666630748));
#23389=CARTESIAN_POINT('Ctrl Pts',(2.56424349027146,-0.522062886964902,
6.50008215105946));
#23390=CARTESIAN_POINT('Ctrl Pts',(2.55232465369528,-0.410425773087965,
6.73782039475945));
#23391=CARTESIAN_POINT('Ctrl Pts',(2.54040581711911,-0.19858907062663,6.89308342832313));
#23392=CARTESIAN_POINT('Ctrl Pts',(2.52848698054292,0.0617246536500735,
6.92797742227401));
#23393=CARTESIAN_POINT('Ctrl Pts',(2.51656814396674,0.306971377021502,6.8339796336226));
#23394=CARTESIAN_POINT('Ctrl Pts',(2.50464930739056,0.477279320739804,6.63403891232169));
#23395=CARTESIAN_POINT('Ctrl Pts',(2.49273047081439,0.531073600862929,6.3769640630774));
#23396=CARTESIAN_POINT('Ctrl Pts',(2.48081163423821,0.455221493256117,6.12551290982166));
#23397=CARTESIAN_POINT('Ctrl Pts',(2.46889279766203,0.268240284898955,5.94106977614238));
#23398=CARTESIAN_POINT('Ctrl Pts',(2.45697396108585,0.0157759417689948,
5.86866121228054));
#23399=CARTESIAN_POINT('Ctrl Pts',(2.44505512450967,-0.240539628301038,
5.92596363104932));
#23400=CARTESIAN_POINT('Ctrl Pts',(2.43313628793349,-0.438134411540293,
6.09898832463164));
#23401=CARTESIAN_POINT('Ctrl Pts',(2.42121745135731,-0.528771348081292,
6.34549630925116));
#23402=CARTESIAN_POINT('Ctrl Pts',(2.40929861478113,-0.490324055555984,
6.60530979488368));
#23403=CARTESIAN_POINT('Ctrl Pts',(2.39737977820495,-0.332178326477852,
6.81500283186379));
#23404=CARTESIAN_POINT('Ctrl Pts',(2.38546094162877,-0.092940867251264,
6.92338493135519));
#23405=CARTESIAN_POINT('Ctrl Pts',(2.37354210505259,0.168985416607936,6.90399773818908));
#23406=CARTESIAN_POINT('Ctrl Pts',(2.36162326847641,0.38965879870384,6.76157407502307));
#23407=CARTESIAN_POINT('Ctrl Pts',(2.34970443190023,0.515208255680234,6.5308825596382));
#23408=CARTESIAN_POINT('Ctrl Pts',(2.33778559532405,0.514984518987432,6.26823985300105));
#23409=CARTESIAN_POINT('Ctrl Pts',(2.32586675874787,0.389042207488899,6.03776257519368));
#23410=CARTESIAN_POINT('Ctrl Pts',(2.31394792217169,0.168126493747137,5.89571508724314));
#23411=CARTESIAN_POINT('Ctrl Pts',(2.30202908559551,-0.0938324405162212,
5.87677417471489));
#23412=CARTESIAN_POINT('Ctrl Pts',(2.29011024901934,-0.332884898468083,
5.98556371357228));
#23413=CARTESIAN_POINT('Ctrl Pts',(2.27819141244316,-0.490673136844557,
6.19552588451105));
#23414=CARTESIAN_POINT('Ctrl Pts',(2.26627257586698,-0.528677721240565,
6.45540449655913));
#23415=CARTESIAN_POINT('Ctrl Pts',(2.2543537392908,-0.437620931409163,6.70175770318116));
#23416=CARTESIAN_POINT('Ctrl Pts',(2.24243490271462,-0.239731649313908,
6.87444549491937));
#23417=CARTESIAN_POINT('Ctrl Pts',(2.23051606613844,0.0166811816108265,
6.93131114145764));
#23418=CARTESIAN_POINT('Ctrl Pts',(2.21859722956226,0.269021783055123,6.85847254173578));
#23419=CARTESIAN_POINT('Ctrl Pts',(2.20667839298608,0.455688500581004,6.67371112931225));
#23420=CARTESIAN_POINT('Ctrl Pts',(2.1947595564099,0.53111204424701,6.42213106706975));
#23421=CARTESIAN_POINT('Ctrl Pts',(2.18284071983372,0.476879959029563,6.1651483330086));
#23422=CARTESIAN_POINT('Ctrl Pts',(2.17092188325754,0.306231393425269,5.96549786619889));
#23423=CARTESIAN_POINT('Ctrl Pts',(2.15900304668136,0.0608253588918372,
5.8719184725451));
#23424=CARTESIAN_POINT('Ctrl Pts',(2.14708421010518,-0.199429574813985,
5.90725502825896));
#23425=CARTESIAN_POINT('Ctrl Pts',(2.135165373529,-0.410999230249818,6.06288076079265));
#23426=CARTESIAN_POINT('Ctrl Pts',(2.12324653695282,-0.522235994732442,
6.30080495423084));
#23427=CARTESIAN_POINT('Ctrl Pts',(2.11132770037665,-0.505982491766854,
6.56294356165447));
#23428=CARTESIAN_POINT('Ctrl Pts',(2.09940886380046,-0.366211204665212,
6.78530674521469));
#23429=CARTESIAN_POINT('Ctrl Pts',(2.08749002722428,-0.137033499838515,
6.91360287657764));
#23430=CARTESIAN_POINT('Ctrl Pts',(2.07557119064811,0.125581190928044,6.91652919922544));
#23431=CARTESIAN_POINT('Ctrl Pts',(2.06365235407193,0.357565218298462,6.79333282215497));
#23432=CARTESIAN_POINT('Ctrl Pts',(2.05570646302114,0.453961018087142,6.64722068416873));
#23433=CARTESIAN_POINT('Ctrl Pts',(2.05173351749575,0.481760682217403,6.56704686488953));
#23434=CARTESIAN_POINT('Ctrl Pts',(2.61608882750142,-0.12505876634041,5.9344718704462));
#23435=CARTESIAN_POINT('Ctrl Pts',(2.61211588197602,-0.202531190940192,
5.95528394436993));
#23436=CARTESIAN_POINT('Ctrl Pts',(2.60416999092524,-0.346801290927786,
6.03633599705392));
#23437=CARTESIAN_POINT('Ctrl Pts',(2.59225115434906,-0.478597955464431,
6.24678417477103));
#23438=CARTESIAN_POINT('Ctrl Pts',(2.58033231777288,-0.493531503458158,
6.49461253752179));
#23439=CARTESIAN_POINT('Ctrl Pts',(2.5684134811967,-0.387995496151209,6.71935809169225));
#23440=CARTESIAN_POINT('Ctrl Pts',(2.55649464462052,-0.187735931903752,
6.86613580813106));
#23441=CARTESIAN_POINT('Ctrl Pts',(2.54457580804434,0.0583513248632879,
6.89912280208567));
#23442=CARTESIAN_POINT('Ctrl Pts',(2.53265697146816,0.290195010989602,6.81026210902899));
#23443=CARTESIAN_POINT('Ctrl Pts',(2.52073813489198,0.451195414605367,6.62124839583474));
#23444=CARTESIAN_POINT('Ctrl Pts',(2.5088192983158,0.50204977067914,6.37822300556726));
#23445=CARTESIAN_POINT('Ctrl Pts',(2.49690046173962,0.430343074719011,6.14051396933589));
#23446=CARTESIAN_POINT('Ctrl Pts',(2.48498162516344,0.253580621031822,5.96615088140125));
#23447=CARTESIAN_POINT('Ctrl Pts',(2.47306278858726,0.0149137670080035,
5.89769953525455));
#23448=CARTESIAN_POINT('Ctrl Pts',(2.46114395201109,-0.227393839632693,
5.95187030585109));
#23449=CARTESIAN_POINT('Ctrl Pts',(2.44922511543491,-0.414189823186519,
6.11543898558529));
#23450=CARTESIAN_POINT('Ctrl Pts',(2.43730627885873,-0.499873338864062,
6.34847500347002));
#23451=CARTESIAN_POINT('Ctrl Pts',(2.42538744228255,-0.463527238503961,
6.59408936025449));
#23452=CARTESIAN_POINT('Ctrl Pts',(2.41346860570637,-0.314024369431667,
6.79232241299485));
#23453=CARTESIAN_POINT('Ctrl Pts',(2.40154976913019,-0.0878615337203718,
6.89478129648476));
#23454=CARTESIAN_POINT('Ctrl Pts',(2.38963093255401,0.159750154250334,6.87645363744213));
#23455=CARTESIAN_POINT('Ctrl Pts',(2.37771209597783,0.368363462643409,6.74181360390328));
#23456=CARTESIAN_POINT('Ctrl Pts',(2.36579325940165,0.487051486264749,6.52372966561601));
#23457=CARTESIAN_POINT('Ctrl Pts',(2.35387442282547,0.486839977059375,6.27544070825967));
#23458=CARTESIAN_POINT('Ctrl Pts',(2.34195558624929,0.367780568902201,6.05755929920087));
#23459=CARTESIAN_POINT('Ctrl Pts',(2.33003674967311,0.158938172587915,5.92327488243597));
#23460=CARTESIAN_POINT('Ctrl Pts',(2.31811791309693,-0.0887043814019138,
5.90536911424148));
#23461=CARTESIAN_POINT('Ctrl Pts',(2.30619907652075,-0.314692326387328,
6.0082131700313));
#23462=CARTESIAN_POINT('Ctrl Pts',(2.29428023994457,-0.463857242067669,
6.20670064822607));
#23463=CARTESIAN_POINT('Ctrl Pts',(2.28236140336839,-0.499784828846167,
6.45237657218681));
#23464=CARTESIAN_POINT('Ctrl Pts',(2.27044256679221,-0.413704405380657,
6.68526627088336));
#23465=CARTESIAN_POINT('Ctrl Pts',(2.25852373021604,-0.226630017698138,
6.84851646087657));
#23466=CARTESIAN_POINT('Ctrl Pts',(2.24660489363986,0.0157695343710637,
6.90227432938608));
#23467=CARTESIAN_POINT('Ctrl Pts',(2.23468605706368,0.254319409345632,6.83341644937185));
#23468=CARTESIAN_POINT('Ctrl Pts',(2.2227672204875,0.430784559515061,6.65875247702062));
#23469=CARTESIAN_POINT('Ctrl Pts',(2.21084838391132,0.502086113084658,6.42092157683831));
#23470=CARTESIAN_POINT('Ctrl Pts',(2.19892954733514,0.450817878507322,6.1779832675451));
#23471=CARTESIAN_POINT('Ctrl Pts',(2.18701071075896,0.289495468413598,5.98924394607454));
#23472=CARTESIAN_POINT('Ctrl Pts',(2.17509187418278,0.05750117767764,5.90077878221055));
#23473=CARTESIAN_POINT('Ctrl Pts',(2.1631730376066,-0.188530501496047,5.93418415137954));
#23474=CARTESIAN_POINT('Ctrl Pts',(2.15125420103042,-0.388537613168766,
6.08130474484033));
#23475=CARTESIAN_POINT('Ctrl Pts',(2.13933536445424,-0.493695150671756,
6.30622608636544));
#23476=CARTESIAN_POINT('Ctrl Pts',(2.12741652787806,-0.478329921778157,
6.55403849415475));
#23477=CARTESIAN_POINT('Ctrl Pts',(2.11549769130188,-0.346197308665989,
6.76424925426879));
#23478=CARTESIAN_POINT('Ctrl Pts',(2.1035788547257,-0.129544449314556,6.88553384311886));
#23479=CARTESIAN_POINT('Ctrl Pts',(2.09166001814953,0.11871802327322,6.88830023860881));
#23480=CARTESIAN_POINT('Ctrl Pts',(2.07974118157334,0.338023836164873,6.77183669616154));
#23481=CARTESIAN_POINT('Ctrl Pts',(2.07179529052256,0.429151486079503,6.63370976752069));
#23482=CARTESIAN_POINT('Ctrl Pts',(2.06782234499716,0.455431864126683,6.55791754678483));
#23483=CARTESIAN_POINT('Ctrl Pts',(2.63217765500284,-0.117829036123926,
5.96138436033673));
#23484=CARTESIAN_POINT('Ctrl Pts',(2.62820470947744,-0.190822728480749,
5.98099327446513));
#23485=CARTESIAN_POINT('Ctrl Pts',(2.62025881842666,-0.326752478313469,
6.05735965423274));
#23486=CARTESIAN_POINT('Ctrl Pts',(2.60833998185048,-0.450929890270581,
6.25564168323458));
#23487=CARTESIAN_POINT('Ctrl Pts',(2.5964211452743,-0.465000119951414,6.48914292398412));
#23488=CARTESIAN_POINT('Ctrl Pts',(2.58450230869812,-0.365565219214455,
6.70089578862506));
#23489=CARTESIAN_POINT('Ctrl Pts',(2.57258347212194,-0.176882793180874,
6.83918818793898));
#23490=CARTESIAN_POINT('Ctrl Pts',(2.56066463554576,0.0549779960765018,
6.87026818189733));
#23491=CARTESIAN_POINT('Ctrl Pts',(2.54874579896958,0.273418644957702,6.78654458443538));
#23492=CARTESIAN_POINT('Ctrl Pts',(2.5368269623934,0.42511150847093,6.60845787934779));
#23493=CARTESIAN_POINT('Ctrl Pts',(2.52490812581722,0.473025940495352,6.37948194805711));
#23494=CARTESIAN_POINT('Ctrl Pts',(2.51298928924104,0.405464656181905,6.15551502885011));
#23495=CARTESIAN_POINT('Ctrl Pts',(2.50107045266486,0.23892095716469,5.99123198666013));
#23496=CARTESIAN_POINT('Ctrl Pts',(2.48915161608868,0.014051592247013,5.92673785822857));
#23497=CARTESIAN_POINT('Ctrl Pts',(2.4772327795125,-0.214248050964349,5.97777698065287));
#23498=CARTESIAN_POINT('Ctrl Pts',(2.46531394293632,-0.390245234832745,
6.13188964653893));
#23499=CARTESIAN_POINT('Ctrl Pts',(2.45339510636014,-0.470975329646833,
6.35145369768889));
#23500=CARTESIAN_POINT('Ctrl Pts',(2.44147626978396,-0.436730421451937,
6.5828689256253));
#23501=CARTESIAN_POINT('Ctrl Pts',(2.42955743320779,-0.295870412385483,
6.76964199412591));
#23502=CARTESIAN_POINT('Ctrl Pts',(2.41763859663161,-0.0827822001894799,
6.86617766161433));
#23503=CARTESIAN_POINT('Ctrl Pts',(2.40571976005543,0.150514891892733,6.84890953669518));
#23504=CARTESIAN_POINT('Ctrl Pts',(2.39380092347925,0.347068126582978,6.7220531327835));
#23505=CARTESIAN_POINT('Ctrl Pts',(2.38188208690307,0.458894716849264,6.51657677159381));
#23506=CARTESIAN_POINT('Ctrl Pts',(2.36996325032689,0.458695435131318,6.28264156351829));
#23507=CARTESIAN_POINT('Ctrl Pts',(2.35804441375071,0.346518930315503,6.07735602320807));
#23508=CARTESIAN_POINT('Ctrl Pts',(2.34612557717453,0.149749851428694,5.9508346776288));
#23509=CARTESIAN_POINT('Ctrl Pts',(2.33420674059835,-0.0835763222876063,
5.93396405376808));
#23510=CARTESIAN_POINT('Ctrl Pts',(2.32228790402217,-0.296499754306572,
6.03086262649031));
#23511=CARTESIAN_POINT('Ctrl Pts',(2.31036906744599,-0.437041347290782,
6.2178754119411));
#23512=CARTESIAN_POINT('Ctrl Pts',(2.29845023086981,-0.470891936451769,
6.44934864781448));
#23513=CARTESIAN_POINT('Ctrl Pts',(2.28653139429363,-0.389787879352151,
6.66877483858555));
#23514=CARTESIAN_POINT('Ctrl Pts',(2.27461255771745,-0.213528386082369,
6.82258742683378));
#23515=CARTESIAN_POINT('Ctrl Pts',(2.26269372114127,0.0148578871313011,
6.87323751731453));
#23516=CARTESIAN_POINT('Ctrl Pts',(2.2507748845651,0.239617035636141,6.80836035700791));
#23517=CARTESIAN_POINT('Ctrl Pts',(2.23885604798891,0.405880618449119,6.64379382472899));
#23518=CARTESIAN_POINT('Ctrl Pts',(2.22693721141274,0.473060181922306,6.41971208660688));
#23519=CARTESIAN_POINT('Ctrl Pts',(2.21501837483656,0.424755797985082,6.1908182020816));
#23520=CARTESIAN_POINT('Ctrl Pts',(2.20309953826038,0.272759543401928,6.01299002595018));
#23521=CARTESIAN_POINT('Ctrl Pts',(2.1911807016842,0.0541769964634428,5.92963909187599));
#23522=CARTESIAN_POINT('Ctrl Pts',(2.17926186510802,-0.17763142817811,5.96111327450012));
#23523=CARTESIAN_POINT('Ctrl Pts',(2.16734302853184,-0.366075996087714,
6.099728728888));
#23524=CARTESIAN_POINT('Ctrl Pts',(2.15542419195566,-0.465154306611069,
6.31164721850004));
#23525=CARTESIAN_POINT('Ctrl Pts',(2.14350535537948,-0.450677351789461,
6.54513342665504));
#23526=CARTESIAN_POINT('Ctrl Pts',(2.1315865188033,-0.326183412666766,6.74319176332289));
#23527=CARTESIAN_POINT('Ctrl Pts',(2.11966768222712,-0.122055398790597,
6.85746480966008));
#23528=CARTESIAN_POINT('Ctrl Pts',(2.10774884565094,0.111854855618396,6.8600712779922));
#23529=CARTESIAN_POINT('Ctrl Pts',(2.09583000907476,0.318482454031284,6.7503405701681));
#23530=CARTESIAN_POINT('Ctrl Pts',(2.08788411802398,0.404341954071864,6.62019885087265));
#23531=CARTESIAN_POINT('Ctrl Pts',(2.08391117249858,0.429103046035963,6.54878822868013));
#23532=CARTESIAN_POINT('Ctrl Pts',(2.64826648250425,-0.110599305907441,
5.98829685022726));
#23533=CARTESIAN_POINT('Ctrl Pts',(2.64429353697886,-0.179114266021306,
6.00670260456034));
#23534=CARTESIAN_POINT('Ctrl Pts',(2.63634764592807,-0.306703665699153,
6.07838331141156));
#23535=CARTESIAN_POINT('Ctrl Pts',(2.6244288093519,-0.423261825076731,6.26449919169813));
#23536=CARTESIAN_POINT('Ctrl Pts',(2.61250997277572,-0.436468736444671,
6.48367331044645));
#23537=CARTESIAN_POINT('Ctrl Pts',(2.60059113619953,-0.3431349422777,6.68243348555786));
#23538=CARTESIAN_POINT('Ctrl Pts',(2.58867229962336,-0.166029654457996,
6.81224056774691));
#23539=CARTESIAN_POINT('Ctrl Pts',(2.57675346304718,0.0516046672897163,
6.84141356170898));
#23540=CARTESIAN_POINT('Ctrl Pts',(2.564834626471,0.256642278925802,6.76282705984177));
#23541=CARTESIAN_POINT('Ctrl Pts',(2.55291578989482,0.399027602336494,6.59566736286083));
#23542=CARTESIAN_POINT('Ctrl Pts',(2.54099695331864,0.444002110311564,6.38074089054697));
#23543=CARTESIAN_POINT('Ctrl Pts',(2.52907811674246,0.380586237644799,6.17051608836433));
#23544=CARTESIAN_POINT('Ctrl Pts',(2.51715928016628,0.224261293297557,6.016313091919));
#23545=CARTESIAN_POINT('Ctrl Pts',(2.5052404435901,0.0131894174860218,5.95577618120258));
#23546=CARTESIAN_POINT('Ctrl Pts',(2.49332160701392,-0.201102262296004,
6.00368365545465));
#23547=CARTESIAN_POINT('Ctrl Pts',(2.48140277043774,-0.366300646478971,
6.14834030749258));
#23548=CARTESIAN_POINT('Ctrl Pts',(2.46948393386156,-0.442077320429603,
6.35443239190776));
#23549=CARTESIAN_POINT('Ctrl Pts',(2.45756509728538,-0.409933604399914,
6.57164849099611));
#23550=CARTESIAN_POINT('Ctrl Pts',(2.4456462607092,-0.277716455339298,6.74696157525698));
#23551=CARTESIAN_POINT('Ctrl Pts',(2.43372742413302,-0.0777028666585877,
6.8375740267439));
#23552=CARTESIAN_POINT('Ctrl Pts',(2.42180858755684,0.141279629535131,6.82136543594824));
#23553=CARTESIAN_POINT('Ctrl Pts',(2.40988975098066,0.325772790522547,6.70229266166372));
#23554=CARTESIAN_POINT('Ctrl Pts',(2.39797091440449,0.430737947433779,6.50942387757162));
#23555=CARTESIAN_POINT('Ctrl Pts',(2.38605207782831,0.43055089320326,6.28984241877691));
#23556=CARTESIAN_POINT('Ctrl Pts',(2.37413324125213,0.325257291728805,6.09715274721527));
#23557=CARTESIAN_POINT('Ctrl Pts',(2.36221440467595,0.140561530269473,5.97839447282163));
#23558=CARTESIAN_POINT('Ctrl Pts',(2.35029556809977,-0.0784482631732989,
5.96255899329468));
#23559=CARTESIAN_POINT('Ctrl Pts',(2.33837673152359,-0.278307182225817,
6.05351208294933));
#23560=CARTESIAN_POINT('Ctrl Pts',(2.32645789494741,-0.410225452513894,
6.22905017565613));
#23561=CARTESIAN_POINT('Ctrl Pts',(2.31453905837123,-0.44199904405737,6.44632072344216));
#23562=CARTESIAN_POINT('Ctrl Pts',(2.30262022179505,-0.365871353323644,
6.65228340628776));
#23563=CARTESIAN_POINT('Ctrl Pts',(2.29070138521887,-0.200426754466599,
6.79665839279099));
#23564=CARTESIAN_POINT('Ctrl Pts',(2.27878254864269,0.0139462398915382,
6.84420070524297));
#23565=CARTESIAN_POINT('Ctrl Pts',(2.26686371206651,0.22491466192665,6.78330426464398));
#23566=CARTESIAN_POINT('Ctrl Pts',(2.25494487549033,0.380976677383177,6.62883517243736));
#23567=CARTESIAN_POINT('Ctrl Pts',(2.24302603891415,0.444034250759953,6.41850259637544));
#23568=CARTESIAN_POINT('Ctrl Pts',(2.23110720233797,0.398693717462841,6.2036531366181));
#23569=CARTESIAN_POINT('Ctrl Pts',(2.2191883657618,0.256023618390257,6.03673610582583));
#23570=CARTESIAN_POINT('Ctrl Pts',(2.20726952918561,0.0508528152492455,
5.95849940154143));
#23571=CARTESIAN_POINT('Ctrl Pts',(2.19535069260944,-0.166732354860172,
5.9880423976207));
#23572=CARTESIAN_POINT('Ctrl Pts',(2.18343185603326,-0.343614379006663,
6.11815271293568));
#23573=CARTESIAN_POINT('Ctrl Pts',(2.17151301945708,-0.436613462550383,
6.31706835063465));
#23574=CARTESIAN_POINT('Ctrl Pts',(2.1595941828809,-0.423024781800764,6.53622835915532));
#23575=CARTESIAN_POINT('Ctrl Pts',(2.14767534630472,-0.306169516667542,
6.72213427237698));
#23576=CARTESIAN_POINT('Ctrl Pts',(2.13575650972854,-0.114566348266639,
6.8293957762013));
#23577=CARTESIAN_POINT('Ctrl Pts',(2.12383767315236,0.104991687963572,6.83184231737557));
#23578=CARTESIAN_POINT('Ctrl Pts',(2.11191883657618,0.298941071897694,6.72884444417467));
#23579=CARTESIAN_POINT('Ctrl Pts',(2.10397294552539,0.379532422064226,6.60668793422461));
#23580=CARTESIAN_POINT('Ctrl Pts',(2.1,0.402774227945242,6.53965891057542));
#23581=CARTESIAN_POINT('Ctrl Pts',(2.1,0.402774227945242,6.53965891057542));
#23582=CARTESIAN_POINT('Ctrl Pts',(2.1,0.398484638758285,6.55741240483299));
#23583=CARTESIAN_POINT('Ctrl Pts',(2.1,0.393037299189535,6.57484669319261));
#23584=CARTESIAN_POINT('Ctrl Pts',(2.1,0.386509552509357,6.59187123411703));
#23585=CARTESIAN_POINT('Ctrl Pts',(2.1,0.381753507363848,6.60427512924121));
#23586=CARTESIAN_POINT('Ctrl Pts',(2.1,0.376423475271725,6.61646161573661));
#23587=CARTESIAN_POINT('Ctrl Pts',(2.1,0.370542725187782,6.62839523023791));
#23588=CARTESIAN_POINT('Ctrl Pts',(2.1,0.367213725298235,6.63515066122709));
#23589=CARTESIAN_POINT('Ctrl Pts',(2.1,0.363707525435473,6.6418256648993));
#23590=CARTESIAN_POINT('Ctrl Pts',(2.1,0.360036351586671,6.64839942538541));
#23591=CARTESIAN_POINT('Ctrl Pts',(2.1,0.35176296808893,6.66321409877431));
#23592=CARTESIAN_POINT('Ctrl Pts',(2.1,0.342644371178579,6.67753242868165));
#23593=CARTESIAN_POINT('Ctrl Pts',(2.1,0.332730966942087,6.69128302674014));
#23594=CARTESIAN_POINT('Ctrl Pts',(2.1,0.326097681493147,6.70048386631449));
#23595=CARTESIAN_POINT('Ctrl Pts',(2.1,0.319108257560132,6.70943048957354));
#23596=CARTESIAN_POINT('Ctrl Pts',(2.1,0.311774677324918,6.7181003705903));
#23597=CARTESIAN_POINT('Ctrl Pts',(2.1,0.308148267079993,6.7223875733389));
#23598=CARTESIAN_POINT('Ctrl Pts',(2.1,0.304437253383367,6.7266073471557));
#23599=CARTESIAN_POINT('Ctrl Pts',(2.1,0.30065086413981,6.73074867775903));
#23600=CARTESIAN_POINT('Ctrl Pts',(2.1,0.284450150446919,6.74846806873983));
#23601=CARTESIAN_POINT('Ctrl Pts',(2.1,0.26684239953173,6.76479115222895));
#23602=CARTESIAN_POINT('Ctrl Pts',(2.1,0.24806300232608,6.77963444611442));
#23603=CARTESIAN_POINT('Ctrl Pts',(2.1,0.229015002355758,6.79469004445943));
#23604=CARTESIAN_POINT('Ctrl Pts',(2.1,0.208760629118366,6.80822418203225));
#23605=CARTESIAN_POINT('Ctrl Pts',(2.1,0.187501868003905,6.82011881527523));
#23606=CARTESIAN_POINT('Ctrl Pts',(2.1,0.182121127272195,6.8231294299218));
#23607=CARTESIAN_POINT('Ctrl Pts',(2.1,0.176675868974013,6.82603481851803));
#23608=CARTESIAN_POINT('Ctrl Pts',(2.1,0.171169051786272,6.82883264150109));
#23609=CARTESIAN_POINT('Ctrl Pts',(2.1,0.165595855256536,6.83166418952754));
#23610=CARTESIAN_POINT('Ctrl Pts',(2.1,0.159966248284264,6.83438207494035));
#23611=CARTESIAN_POINT('Ctrl Pts',(2.1,0.154290568068188,6.83698163141168));
#23612=CARTESIAN_POINT('Ctrl Pts',(2.1,0.139973144289019,6.84353925097815));
#23613=CARTESIAN_POINT('Ctrl Pts',(2.1,0.1253500812197,6.84935087179354));
#23614=CARTESIAN_POINT('Ctrl Pts',(2.1,0.110478871969928,6.85439100862466));
#23615=CARTESIAN_POINT('Ctrl Pts',(2.1,0.091606231881728,6.86078730678786));
#23616=CARTESIAN_POINT('Ctrl Pts',(2.1,0.0723341026865624,6.8659419398207));
#23617=CARTESIAN_POINT('Ctrl Pts',(2.1,0.0527866493565085,6.86986556285165));
#23618=CARTESIAN_POINT('Ctrl Pts',(2.1,0.0364584381349322,6.87314301002196));
#23619=CARTESIAN_POINT('Ctrl Pts',(2.1,0.0199377431301133,6.87556121981262));
#23620=CARTESIAN_POINT('Ctrl Pts',(2.1,0.00329277923049777,6.87711561177094));
#23621=CARTESIAN_POINT('Ctrl Pts',(2.1,-0.00380833581134274,6.87777875025432));
#23622=CARTESIAN_POINT('Ctrl Pts',(2.1,-0.010934154274537,6.87828439261757));
#23623=CARTESIAN_POINT('Ctrl Pts',(2.1,-0.0180564268157742,6.87863124049195));
#23624=CARTESIAN_POINT('Ctrl Pts',(2.1,-0.0436614570733077,6.87987818102488));
#23625=CARTESIAN_POINT('Ctrl Pts',(2.1,-0.0692830486968658,6.87908401838085));
#23626=CARTESIAN_POINT('Ctrl Pts',(2.1,-0.0946701039420577,6.87627112264398));
#23627=CARTESIAN_POINT('Ctrl Pts',(2.1,-0.105116630998588,6.87511364332475));
#23628=CARTESIAN_POINT('Ctrl Pts',(2.1,-0.115523671677657,6.87361376587106));
#23629=CARTESIAN_POINT('Ctrl Pts',(2.1,-0.125874323021446,6.87177056809269));
#23630=CARTESIAN_POINT('Ctrl Pts',(2.1,-0.138413824297786,6.86953758969098));
#23631=CARTESIAN_POINT('Ctrl Pts',(2.1,-0.150870601134534,6.86680082502239));
#23632=CARTESIAN_POINT('Ctrl Pts',(2.1,-0.163219456840939,6.86357425405869));
#23633=CARTESIAN_POINT('Ctrl Pts',(2.1,-0.170695776276485,6.8616208038136));
#23634=CARTESIAN_POINT('Ctrl Pts',(2.1,-0.178132534318461,6.85948775559199));
#23635=CARTESIAN_POINT('Ctrl Pts',(2.1,-0.185524032856684,6.85717764382782));
#23636=CARTESIAN_POINT('Ctrl Pts',(2.1,-0.191333634449564,6.85536193231609));
#23637=CARTESIAN_POINT('Ctrl Pts',(2.1,-0.197115271577026,6.85343663586951));
#23638=CARTESIAN_POINT('Ctrl Pts',(2.1,-0.202852164838079,6.85140831852427));
#23639=CARTESIAN_POINT('Ctrl Pts',(2.1,-0.227408324506361,6.84272632248192));
#23640=CARTESIAN_POINT('Ctrl Pts',(2.1,-0.251209399850707,6.83214163505072));
#23641=CARTESIAN_POINT('Ctrl Pts',(2.1,-0.274050638756253,6.81980030995607));
#23642=CARTESIAN_POINT('Ctrl Pts',(2.1,-0.297081928279728,6.80735629881755));
#23643=CARTESIAN_POINT('Ctrl Pts',(2.1,-0.319138676313367,6.79312590368834));
#23644=CARTESIAN_POINT('Ctrl Pts',(2.1,-0.33999937244817,6.77720843590635));
#23645=CARTESIAN_POINT('Ctrl Pts',(2.1,-0.343569976374306,6.77448393560256));
#23646=CARTESIAN_POINT('Ctrl Pts',(2.1,-0.347105483833496,6.77170989850117));
#23647=CARTESIAN_POINT('Ctrl Pts',(2.1,-0.350604705166974,6.76888668926355));
#23648=CARTESIAN_POINT('Ctrl Pts',(2.1,-0.353884815611532,6.76624026103711));
#23649=CARTESIAN_POINT('Ctrl Pts',(2.1,-0.357133041678995,6.76355062538503));
#23650=CARTESIAN_POINT('Ctrl Pts',(2.1,-0.360348823959175,6.76081852140068));
#23651=CARTESIAN_POINT('Ctrl Pts',(2.46703183294109,-0.426306423912841,
6.39998913682467));
#23652=CARTESIAN_POINT('Ctrl Pts',(2.46387625438919,-0.426248106936643,
6.45633454115753));
#23653=CARTESIAN_POINT('Ctrl Pts',(2.46072067583729,-0.415012427400236,
6.51270250838063));
#23654=CARTESIAN_POINT('Ctrl Pts',(2.45756509728538,-0.39325469889476,6.56466465519153));
#23655=CARTESIAN_POINT('Ctrl Pts',(2.45359215175999,-0.365861221379708,
6.63008618574973));
#23656=CARTESIAN_POINT('Ctrl Pts',(2.4496192062346,-0.321788838359503,6.68852388050336));
#23657=CARTESIAN_POINT('Ctrl Pts',(2.4456462607092,-0.266417048735948,6.73284480312799));
#23658=CARTESIAN_POINT('Ctrl Pts',(2.44167331518381,-0.211045259112394,
6.77716572575262));
#23659=CARTESIAN_POINT('Ctrl Pts',(2.43770036965842,-0.144374062885491,
6.80736987624826));
#23660=CARTESIAN_POINT('Ctrl Pts',(2.43372742413302,-0.0745413820730864,
6.8197705196968));
#23661=CARTESIAN_POINT('Ctrl Pts',(2.42975447860763,-0.00470870126068151,
6.83217116314535));
#23662=CARTESIAN_POINT('Ctrl Pts',(2.42578153308224,0.0682854641372245,
6.82676829954679));
#23663=CARTESIAN_POINT('Ctrl Pts',(2.42180858755684,0.135531407000747,6.80422140536676));
#23664=CARTESIAN_POINT('Ctrl Pts',(2.41783564203145,0.202777349864269,6.78167451118673));
#23665=CARTESIAN_POINT('Ctrl Pts',(2.41386269650606,0.264275070193409,6.74198358642523));
#23666=CARTESIAN_POINT('Ctrl Pts',(2.40988975098066,0.312518123176517,6.68999332669579));
#23667=CARTESIAN_POINT('Ctrl Pts',(2.40591680545527,0.360761176159625,6.63800306696635));
#23668=CARTESIAN_POINT('Ctrl Pts',(2.40194385992988,0.395749561796702,6.57371347226898));
#23669=CARTESIAN_POINT('Ctrl Pts',(2.39797091440449,0.413212578910154,6.50497176512118));
#23670=CARTESIAN_POINT('Ctrl Pts',(2.39399796887909,0.430675596023606,6.43623005797338));
#23671=CARTESIAN_POINT('Ctrl Pts',(2.3900250233537,0.430613244613433,6.36303623837515));
#23672=CARTESIAN_POINT('Ctrl Pts',(2.38605207782831,0.413033135329271,6.29432438331576));
#23673=CARTESIAN_POINT('Ctrl Pts',(2.38207913230291,0.395453026045109,6.22561252825636));
#23674=CARTESIAN_POINT('Ctrl Pts',(2.37810618677752,0.360355158886957,6.16138263773582));
#23675=CARTESIAN_POINT('Ctrl Pts',(2.37413324125213,0.312023598397992,6.10947464674327));
#23676=CARTESIAN_POINT('Ctrl Pts',(2.37016029572673,0.263692037909028,6.05756665575072));
#23677=CARTESIAN_POINT('Ctrl Pts',(2.36618735020134,0.20212678408925,6.01798056428618));
#23678=CARTESIAN_POINT('Ctrl Pts',(2.36221440467595,0.1348425249389,5.99554827196608));
#23679=CARTESIAN_POINT('Ctrl Pts',(2.35824145915055,0.0675582657885491,
5.97311597964598));
#23680=CARTESIAN_POINT('Ctrl Pts',(2.35426851362516,-0.00544499869237483,
5.96783748647033));
#23681=CARTESIAN_POINT('Ctrl Pts',(2.35029556809977,-0.0752564507749232,
5.98035708815828));
#23682=CARTESIAN_POINT('Ctrl Pts',(2.34632262257437,-0.145067902857471,
5.99287668984623));
#23683=CARTESIAN_POINT('Ctrl Pts',(2.34234967704898,-0.211687542541645,
6.02319438639778));
#23684=CARTESIAN_POINT('Ctrl Pts',(2.33837673152359,-0.266983740765077,
6.06760958345802));
#23685=CARTESIAN_POINT('Ctrl Pts',(2.33440378599819,-0.322279938988509,
6.11202478051826));
#23686=CARTESIAN_POINT('Ctrl Pts',(2.3304308404728,-0.366252695751201,6.17053747808719));
#23687=CARTESIAN_POINT('Ctrl Pts',(2.32645789494741,-0.393534672723127,
6.236005584836));
#23688=CARTESIAN_POINT('Ctrl Pts',(2.32331587427864,-0.415110738889366,
6.28778131224916));
#23689=CARTESIAN_POINT('Ctrl Pts',(2.32017385360987,-0.4262475506417,6.34390730291496));
#23690=CARTESIAN_POINT('Ctrl Pts',(2.31703183294109,-0.426305653513777,
6.40001091236462));
#23691=CARTESIAN_POINT('Ctrl Pts',(2.6,-0.132288496556895,5.90755938055567));
#23692=CARTESIAN_POINT('Ctrl Pts',(2.6,-0.157089924837099,5.91642640455182));
#23693=CARTESIAN_POINT('Ctrl Pts',(2.6,-0.181088073064976,5.9272189255245));
#23694=CARTESIAN_POINT('Ctrl Pts',(2.6,-0.204091900162786,5.93978802247808));
#23695=CARTESIAN_POINT('Ctrl Pts',(2.6,-0.226981614101412,5.95229476896469));
#23696=CARTESIAN_POINT('Ctrl Pts',(2.6,-0.248887897831876,5.96656143458844));
#23697=CARTESIAN_POINT('Ctrl Pts',(2.6,-0.269590200964406,5.98248076289354));
#23698=CARTESIAN_POINT('Ctrl Pts',(2.6,-0.276528918772376,5.98781638792494));
#23699=CARTESIAN_POINT('Ctrl Pts',(2.6,-0.283332046569503,5.99333793609881));
#23700=CARTESIAN_POINT('Ctrl Pts',(2.6,-0.289990147837974,5.99904209573216));
#23701=CARTESIAN_POINT('Ctrl Pts',(2.6,-0.296028106433828,6.00421496383698));
#23702=CARTESIAN_POINT('Ctrl Pts',(2.6,-0.301949771037903,6.00954116989861));
#23703=CARTESIAN_POINT('Ctrl Pts',(2.6,-0.307727671725424,6.01499858003089));
#23704=CARTESIAN_POINT('Ctrl Pts',(2.6,-0.318182122624537,6.02487313990129));
#23705=CARTESIAN_POINT('Ctrl Pts',(2.6,-0.32817930410564,6.03518740593773));
#23706=CARTESIAN_POINT('Ctrl Pts',(2.6,-0.337684947200095,6.04592058651842));
#23707=CARTESIAN_POINT('Ctrl Pts',(2.6,-0.35463663907465,6.06506138196275));
#23708=CARTESIAN_POINT('Ctrl Pts',(2.6,-0.370027957593029,6.08553349763026));
#23709=CARTESIAN_POINT('Ctrl Pts',(2.6,-0.383735216002276,6.10712564152075));
#23710=CARTESIAN_POINT('Ctrl Pts',(2.6,-0.39189872132373,6.11998507528124));
#23711=CARTESIAN_POINT('Ctrl Pts',(2.6,-0.399464029634324,6.13324224816933));
#23712=CARTESIAN_POINT('Ctrl Pts',(2.6,-0.406396423774992,6.1468545793287));
#23713=CARTESIAN_POINT('Ctrl Pts',(2.6,-0.409857954474058,6.15365158210118));
#23714=CARTESIAN_POINT('Ctrl Pts',(2.6,-0.413162930739684,6.16054073803517));
#23715=CARTESIAN_POINT('Ctrl Pts',(2.6,-0.416296070484027,6.16749212337976));
#23716=CARTESIAN_POINT('Ctrl Pts',(2.6,-0.426533299061843,6.19020509710957));
#23717=CARTESIAN_POINT('Ctrl Pts',(2.6,-0.434966161858725,6.21362881910558));
#23718=CARTESIAN_POINT('Ctrl Pts',(2.6,-0.441477406647537,6.23756556523482));
#23719=CARTESIAN_POINT('Ctrl Pts',(2.6,-0.443239379224161,6.24404295805621));
#23720=CARTESIAN_POINT('Ctrl Pts',(2.6,-0.444860350146518,6.25055797543335));
#23721=CARTESIAN_POINT('Ctrl Pts',(2.6,-0.44633733619218,6.25710677385474));
#23722=CARTESIAN_POINT('Ctrl Pts',(2.6,-0.450544524902758,6.27576099937518));
#23723=CARTESIAN_POINT('Ctrl Pts',(2.6,-0.453584703119787,6.29468965910361));
#23724=CARTESIAN_POINT('Ctrl Pts',(2.6,-0.455444326288054,6.31378084410223));
#23725=CARTESIAN_POINT('Ctrl Pts',(2.6,-0.456025440853221,6.31974665796081));
#23726=CARTESIAN_POINT('Ctrl Pts',(2.6,-0.456491144811005,6.32572830613997));
#23727=CARTESIAN_POINT('Ctrl Pts',(2.6,-0.456840676091559,6.33172224529114));
#23728=CARTESIAN_POINT('Ctrl Pts',(2.6,-0.457162778165346,6.33724581453417));
#23729=CARTESIAN_POINT('Ctrl Pts',(2.6,-0.457385661676131,6.34277019876787));
#23730=CARTESIAN_POINT('Ctrl Pts',(2.6,-0.457509644065614,6.34829248285953));
#23731=CARTESIAN_POINT('Ctrl Pts',(2.6,-0.458052816417877,6.37248585461552));
#23732=CARTESIAN_POINT('Ctrl Pts',(2.6,-0.456701759624391,6.39664121290135));
#23733=CARTESIAN_POINT('Ctrl Pts',(2.6,-0.453453339531317,6.42053138158929));
#23734=CARTESIAN_POINT('Ctrl Pts',(2.6,-0.450523324248874,6.44207987511851));
#23735=CARTESIAN_POINT('Ctrl Pts',(2.6,-0.446048919178311,6.46341331208366));
#23736=CARTESIAN_POINT('Ctrl Pts',(2.6,-0.439994176553064,6.48435098741415));
#23737=CARTESIAN_POINT('Ctrl Pts',(2.6,-0.438094472520504,6.49092028172105));
#23738=CARTESIAN_POINT('Ctrl Pts',(2.6,-0.436038962655861,6.4974504658391));
#23739=CARTESIAN_POINT('Ctrl Pts',(2.6,-0.43382941905493,6.50393615250028));
#23740=CARTESIAN_POINT('Ctrl Pts',(2.6,-0.431714290768034,6.5101447013206));
#23741=CARTESIAN_POINT('Ctrl Pts',(2.6,-0.42946061872238,6.5163046335942));
#23742=CARTESIAN_POINT('Ctrl Pts',(2.6,-0.427072414698455,6.5224077707279));
#23743=CARTESIAN_POINT('Ctrl Pts',(2.6,-0.421492488317325,6.53666746360122));
#23744=CARTESIAN_POINT('Ctrl Pts',(2.6,-0.415176231857449,6.5506245268354));
#23745=CARTESIAN_POINT('Ctrl Pts',(2.6,-0.408152204549093,6.56422236660796));
#23746=CARTESIAN_POINT('Ctrl Pts',(2.6,-0.402591346359437,6.57498765201209));
#23747=CARTESIAN_POINT('Ctrl Pts',(2.6,-0.396586710322636,6.58552771963742));
#23748=CARTESIAN_POINT('Ctrl Pts',(2.6,-0.390149689096489,6.59581166017504));
#23749=CARTESIAN_POINT('Ctrl Pts',(2.6,-0.386403333843806,6.6017969277853));
#23750=CARTESIAN_POINT('Ctrl Pts',(2.6,-0.382511806820547,6.60769294534655));
#23751=CARTESIAN_POINT('Ctrl Pts',(2.6,-0.378483683496843,6.61348517016826));
#23752=CARTESIAN_POINT('Ctrl Pts',(2.6,-0.365269544048599,6.63248639241469));
#23753=CARTESIAN_POINT('Ctrl Pts',(2.6,-0.350570496167934,6.65040177272496));
#23754=CARTESIAN_POINT('Ctrl Pts',(2.6,-0.334470605331163,6.66701291851188));
#23755=CARTESIAN_POINT('Ctrl Pts',(2.6,-0.332980284132811,6.66855056512987));
#23756=CARTESIAN_POINT('Ctrl Pts',(2.6,-0.331477939680677,6.67007700481367));
#23757=CARTESIAN_POINT('Ctrl Pts',(2.6,-0.329963627179693,6.67159204424712));
#23758=CARTESIAN_POINT('Ctrl Pts',(2.6,-0.327462974104075,6.67409389773937));
#23759=CARTESIAN_POINT('Ctrl Pts',(2.6,-0.324929685151723,6.67656466471947));
#23760=CARTESIAN_POINT('Ctrl Pts',(2.6,-0.322364416527274,6.67900379523474));
#23761=CARTESIAN_POINT('Origin',(-2.93123464956316,0.,6.4));
#23762=CARTESIAN_POINT('Ctrl Pts',(-2.55623464956316,0.509888470297935,
6.40001295625876));
#23763=CARTESIAN_POINT('Ctrl Pts',(-2.55512836300704,0.509911167721204,
6.42364295379955));
#23764=CARTESIAN_POINT('Ctrl Pts',(-2.55004913092554,0.502507177574701,
6.53211994282295));
#23765=CARTESIAN_POINT('Ctrl Pts',(-2.54099695331864,0.426919346618493,
6.7167170754366));
#23766=CARTESIAN_POINT('Ctrl Pts',(-2.52907811674246,0.223174193283009,
6.88245524211623));
#23767=CARTESIAN_POINT('Ctrl Pts',(-2.51715928016628,-0.0350524704178637,
6.93041600240246));
#23768=CARTESIAN_POINT('Ctrl Pts',(-2.5052404435901,-0.284722093726431,
6.84889099741939));
#23769=CARTESIAN_POINT('Ctrl Pts',(-2.49332160701392,-0.464885050226796,
6.6577822578485));
#23770=CARTESIAN_POINT('Ctrl Pts',(-2.48140277043774,-0.531559769507257,
6.40374342750432));
#23771=CARTESIAN_POINT('Ctrl Pts',(-2.46948393386156,-0.468469545343797,
6.14879075163119));
#23772=CARTESIAN_POINT('Ctrl Pts',(-2.45756509728538,-0.291016032073294,
5.95516354586177));
#23773=CARTESIAN_POINT('Ctrl Pts',(-2.4456462607092,-0.0425193718295788,
5.87013029471448));
#23774=CARTESIAN_POINT('Ctrl Pts',(-2.43372742413302,0.216357163144678,
5.91444940567057));
#23775=CARTESIAN_POINT('Ctrl Pts',(-2.42180858755684,0.422416354717456,
6.07730165027367));
#23776=CARTESIAN_POINT('Ctrl Pts',(-2.41264432936689,0.501564565860727,
6.26308799447805));
#23777=CARTESIAN_POINT('Ctrl Pts',(-2.40745301670233,0.50990474610345,6.37396275616984));
#23778=CARTESIAN_POINT('Ctrl Pts',(-2.40623464956316,0.509881639433629,
6.39998778127036));
#23779=CARTESIAN_POINT('Ctrl Pts',(-2.56876535043684,0.509867809550215,
6.40001069114481));
#23780=CARTESIAN_POINT('Ctrl Pts',(-2.56725806371505,0.509887058630054,
6.4322090151272));
#23781=CARTESIAN_POINT('Ctrl Pts',(-2.56177783146786,0.498968432159698,
6.54926324266892));
#23782=CARTESIAN_POINT('Ctrl Pts',(-2.55232465369528,0.410425773087965,
6.73782039475945));
#23783=CARTESIAN_POINT('Ctrl Pts',(-2.54040581711911,0.19858907062663,6.89308342832313));
#23784=CARTESIAN_POINT('Ctrl Pts',(-2.52848698054292,-0.0617246536500735,
6.92797742227401));
#23785=CARTESIAN_POINT('Ctrl Pts',(-2.51656814396674,-0.306971377021502,
6.8339796336226));
#23786=CARTESIAN_POINT('Ctrl Pts',(-2.50464930739056,-0.477279320739804,
6.63403891232169));
#23787=CARTESIAN_POINT('Ctrl Pts',(-2.49273047081439,-0.531073600862929,
6.3769640630774));
#23788=CARTESIAN_POINT('Ctrl Pts',(-2.48081163423821,-0.455221493256117,
6.12551290982166));
#23789=CARTESIAN_POINT('Ctrl Pts',(-2.46889279766203,-0.268240284898955,
5.94106977614238));
#23790=CARTESIAN_POINT('Ctrl Pts',(-2.45697396108585,-0.0157759417689948,
5.86866121228054));
#23791=CARTESIAN_POINT('Ctrl Pts',(-2.44505512450967,0.240539628301038,
5.92596363104932));
#23792=CARTESIAN_POINT('Ctrl Pts',(-2.43313628793349,0.438134411540293,
6.09898832463164));
#23793=CARTESIAN_POINT('Ctrl Pts',(-2.42437302990921,0.504774712912163,
6.28023194354175));
#23794=CARTESIAN_POINT('Ctrl Pts',(-2.41958271741033,0.509925751376541,
6.3825301408573));
#23795=CARTESIAN_POINT('Ctrl Pts',(-2.41876535043684,0.509907683680876,
6.3999870064905));
#23796=CARTESIAN_POINT('Ctrl Pts',(-2.6,-0.322335278395778,6.67898325810255));
#23797=CARTESIAN_POINT('Ctrl Pts',(-2.59602705447461,-0.368763212726337,
6.62534075195518));
#23798=CARTESIAN_POINT('Ctrl Pts',(-2.58808116342382,-0.434258099467944,
6.4944682619995));
#23799=CARTESIAN_POINT('Ctrl Pts',(-2.57616232684764,-0.426482264300449,
6.27500430516079));
#23800=CARTESIAN_POINT('Ctrl Pts',(-2.56424349027146,-0.314584469477882,
6.08608472387891));
#23801=CARTESIAN_POINT('Ctrl Pts',(-2.55232465369528,-0.125891708691813,
5.97378227942249));
#23802=CARTESIAN_POINT('Ctrl Pts',(-2.5404058171191,0.0935351747046863,
5.96553560214966));
#23803=CARTESIAN_POINT('Ctrl Pts',(-2.52848698054292,0.290127651295543,
6.06334746928321));
#23804=CARTESIAN_POINT('Ctrl Pts',(-2.51656814396674,0.415894108139653,
6.24334485866553));
#23805=CARTESIAN_POINT('Ctrl Pts',(-2.50464930739057,0.440131934448267,
6.46158434769009));
#23806=CARTESIAN_POINT('Ctrl Pts',(-2.49273047081439,0.356924333130935,
6.66479013386668));
#23807=CARTESIAN_POINT('Ctrl Pts',(-2.48081163423821,0.186583954886344,
6.80335491216739));
#23808=CARTESIAN_POINT('Ctrl Pts',(-2.46889279766203,-0.0293054876233287,
6.8434523275626));
#23809=CARTESIAN_POINT('Ctrl Pts',(-2.45697396108585,-0.238040848314528,
6.77529365012726));
#23810=CARTESIAN_POINT('Ctrl Pts',(-2.44505512450967,-0.388665418536347,
6.61551789864839));
#23811=CARTESIAN_POINT('Ctrl Pts',(-2.43313628793349,-0.444408569799851,
6.40312967865285));
#23812=CARTESIAN_POINT('Ctrl Pts',(-2.42121745135731,-0.391662222357444,
6.18997744149907));
#23813=CARTESIAN_POINT('Ctrl Pts',(-2.40929861478113,-0.243302872078535,
6.0280961357146));
#23814=CARTESIAN_POINT('Ctrl Pts',(-2.39737977820495,-0.0355481627984888,
5.95700440211175));
#23815=CARTESIAN_POINT('Ctrl Pts',(-2.38546094162877,0.180884602174105,
5.99405723011839));
#23816=CARTESIAN_POINT('Ctrl Pts',(-2.37354210505259,0.353159623487059,
6.13020924399229));
#23817=CARTESIAN_POINT('Ctrl Pts',(-2.36162326847641,0.439220937561425,
6.33222286740014));
#23818=CARTESIAN_POINT('Ctrl Pts',(-2.34970443190023,0.418059163834771,
6.55078231736932));
#23819=CARTESIAN_POINT('Ctrl Pts',(-2.33778559532405,0.29484033726761,6.73253262578912));
#23820=CARTESIAN_POINT('Ctrl Pts',(-2.32586675874787,0.099644770368915,
6.83310471186003));
#23821=CARTESIAN_POINT('Ctrl Pts',(-2.3139479221717,-0.119876185075048,
6.82794680971604));
#23822=CARTESIAN_POINT('Ctrl Pts',(-2.30202908559551,-0.310132837249173,
6.71831807199288));
#23823=CARTESIAN_POINT('Ctrl Pts',(-2.29011024901934,-0.424679527547163,
6.53098118406136));
#23824=CARTESIAN_POINT('Ctrl Pts',(-2.27819141244315,-0.435552994685514,
6.31166902859576));
#23825=CARTESIAN_POINT('Ctrl Pts',(-2.26627257586698,-0.340098796199685,
6.11392032482827));
#23826=CARTESIAN_POINT('Ctrl Pts',(-2.2543537392908,-0.16161931364965,5.98600969928979));
#23827=CARTESIAN_POINT('Ctrl Pts',(-2.24243490271462,0.0563148495252739,
5.95916283101918));
#23828=CARTESIAN_POINT('Ctrl Pts',(-2.23051606613844,0.260501371261513,
6.03993360741091));
#23829=CARTESIAN_POINT('Ctrl Pts',(-2.21859722956226,0.401094017530737,
6.20860417742001));
#23830=CARTESIAN_POINT('Ctrl Pts',(-2.20667839298608,0.44377116171621,6.42399850480546));
#23831=CARTESIAN_POINT('Ctrl Pts',(-2.1947595564099,0.378114410354912,6.63353428436548));
#23832=CARTESIAN_POINT('Ctrl Pts',(-2.18284071983372,0.220151966921295,
6.78605943828148));
#23833=CARTESIAN_POINT('Ctrl Pts',(-2.17092188325754,0.00844577862671016,
6.84433931427905));
#23834=CARTESIAN_POINT('Ctrl Pts',(-2.15900304668136,-0.205322181057602,
6.79414666881739));
#23835=CARTESIAN_POINT('Ctrl Pts',(-2.14708421010518,-0.368966714730599,
6.64773436383049));
#23836=CARTESIAN_POINT('Ctrl Pts',(-2.135165373529,-0.442538599255273,6.44084520364718));
#23837=CARTESIAN_POINT('Ctrl Pts',(-2.12324653695282,-0.408077698331108,
6.22398416943617));
#23838=CARTESIAN_POINT('Ctrl Pts',(-2.11132770037664,-0.273995984823229,
6.05009380941852));
#23839=CARTESIAN_POINT('Ctrl Pts',(-2.09940886380046,-0.0730271011145798,
5.96161967407919));
#23840=CARTESIAN_POINT('Ctrl Pts',(-2.08749002722429,0.145771140848075,
5.98017031606292));
#23841=CARTESIAN_POINT('Ctrl Pts',(-2.07557119064811,0.328978055262558,
6.10119490525287));
#23842=CARTESIAN_POINT('Ctrl Pts',(-2.06365235407193,0.431879950098104,
6.29519514237415));
#23843=CARTESIAN_POINT('Ctrl Pts',(-2.05570646302114,0.430162668703658,
6.44153119316515));
#23844=CARTESIAN_POINT('Ctrl Pts',(-2.05173351749575,0.411845039474987,
6.51006976632957));
#23845=CARTESIAN_POINT('Ctrl Pts',(-2.61608882750142,-0.34340590883904,
6.69722002436839));
#23846=CARTESIAN_POINT('Ctrl Pts',(-2.61211588197602,-0.392868775775771,
6.64007097860578));
#23847=CARTESIAN_POINT('Ctrl Pts',(-2.60416999092524,-0.462644976561947,
6.5006435272299));
#23848=CARTESIAN_POINT('Ctrl Pts',(-2.59225115434906,-0.454360845343155,
6.26683350205768));
#23849=CARTESIAN_POINT('Ctrl Pts',(-2.58033231777288,-0.335148439802654,
6.065564497838));
#23850=CARTESIAN_POINT('Ctrl Pts',(-2.5684134811967,-0.134121083034322,
5.94592099125275));
#23851=CARTESIAN_POINT('Ctrl Pts',(-2.55649464462052,0.0996494452538391,
5.9371352396035));
#23852=CARTESIAN_POINT('Ctrl Pts',(-2.54457580804434,0.309092911791522,
6.04134093900881));
#23853=CARTESIAN_POINT('Ctrl Pts',(-2.53265697146816,0.443080555430665,
6.23310451945562));
#23854=CARTESIAN_POINT('Ctrl Pts',(-2.52073813489198,0.468902776359187,
6.46561003497361));
#23855=CARTESIAN_POINT('Ctrl Pts',(-2.5088192983158,0.380256004293454,6.68209911438999));
#23856=CARTESIAN_POINT('Ctrl Pts',(-2.49690046173962,0.198780701018566,
6.829721688817));
#23857=CARTESIAN_POINT('Ctrl Pts',(-2.48498162516344,-0.0312211485548406,
6.87244021917589));
#23858=CARTESIAN_POINT('Ctrl Pts',(-2.47306278858727,-0.253601263451829,
6.79982609922463));
#23859=CARTESIAN_POINT('Ctrl Pts',(-2.46114395201108,-0.414071962433164,
6.62960601838176));
#23860=CARTESIAN_POINT('Ctrl Pts',(-2.44922511543491,-0.473458969702319,
6.40333426160334));
#23861=CARTESIAN_POINT('Ctrl Pts',(-2.43730627885873,-0.417264663352895,
6.17624854487645));
#23862=CARTESIAN_POINT('Ctrl Pts',(-2.42538744228255,-0.259207258743454,
6.00378527243032));
#23863=CARTESIAN_POINT('Ctrl Pts',(-2.41346860570637,-0.0378718991421855,
5.92804636631267));
#23864=CARTESIAN_POINT('Ctrl Pts',(-2.40154976913019,0.192708789164296,
5.96752128863578));
#23865=CARTESIAN_POINT('Ctrl Pts',(-2.38963093255401,0.376245200563858,
6.11257337941941));
#23866=CARTESIAN_POINT('Ctrl Pts',(-2.37771209597783,0.467932228811824,
6.32779236596503));
#23867=CARTESIAN_POINT('Ctrl Pts',(-2.36579325940165,0.445387137950485,
6.56063875785105));
#23868=CARTESIAN_POINT('Ctrl Pts',(-2.35387442282547,0.314113659806958,
6.75426984333229));
#23869=CARTESIAN_POINT('Ctrl Pts',(-2.34195558624929,0.106158417098793,
6.86141619353295));
#23870=CARTESIAN_POINT('Ctrl Pts',(-2.33003674967311,-0.127712332602043,
6.85592112615381));
#23871=CARTESIAN_POINT('Ctrl Pts',(-2.31811791309693,-0.330405810268198,
6.73912610297154));
#23872=CARTESIAN_POINT('Ctrl Pts',(-2.30619907652075,-0.452440266074759,
6.53954325067136));
#23873=CARTESIAN_POINT('Ctrl Pts',(-2.29428023994457,-0.464024517365714,
6.30589494992706));
#23874=CARTESIAN_POINT('Ctrl Pts',(-2.28236140336839,-0.362330604286552,
6.09521967517282));
#23875=CARTESIAN_POINT('Ctrl Pts',(-2.27044256679221,-0.172184154232268,
5.95894770137019));
#23876=CARTESIAN_POINT('Ctrl Pts',(-2.25852373021603,0.0599960766894875,
5.93034588886046));
#23877=CARTESIAN_POINT('Ctrl Pts',(-2.24660489363985,0.277530001050755,
6.01639654398105));
#23878=CARTESIAN_POINT('Ctrl Pts',(-2.23468605706368,0.427313002490913,
6.19609288586657));
#23879=CARTESIAN_POINT('Ctrl Pts',(-2.2227672204875,0.472779895096048,6.42556725529552));
#23880=CARTESIAN_POINT('Ctrl Pts',(-2.21084838391132,0.402831248814268,
6.64880011138319));
#23881=CARTESIAN_POINT('Ctrl Pts',(-2.19892954733514,0.234543009563112,
6.81129563269882));
#23882=CARTESIAN_POINT('Ctrl Pts',(-2.18701071075896,0.00899786799506803,
6.8733851870398));
#23883=CARTESIAN_POINT('Ctrl Pts',(-2.17509187418278,-0.218743820229089,
6.81991151478903));
#23884=CARTESIAN_POINT('Ctrl Pts',(-2.1631730376066,-0.393085580436657,
6.66392843124485));
#23885=CARTESIAN_POINT('Ctrl Pts',(-2.15125420103042,-0.471466761658698,
6.44351520053897));
#23886=CARTESIAN_POINT('Ctrl Pts',(-2.13933536445424,-0.43475319726025,
6.2124782476009));
#23887=CARTESIAN_POINT('Ctrl Pts',(-2.12741652787806,-0.291906739636914,
6.02722090494389));
#23888=CARTESIAN_POINT('Ctrl Pts',(-2.11549769130188,-0.0778007860416099,
5.93296333249894));
#23889=CARTESIAN_POINT('Ctrl Pts',(-2.1035788547257,0.155300007354369,5.95272660539192));
#23890=CARTESIAN_POINT('Ctrl Pts',(-2.09166001814952,0.350482915235934,
6.08166241176561));
#23891=CARTESIAN_POINT('Ctrl Pts',(-2.07974118157334,0.46011137071598,6.28834418757117));
#23892=CARTESIAN_POINT('Ctrl Pts',(-2.07179529052256,0.458281832910106,
6.44424603228361));
#23893=CARTESIAN_POINT('Ctrl Pts',(-2.06782234499716,0.438766804507522,
6.51726488124485));
#23894=CARTESIAN_POINT('Ctrl Pts',(-2.63217765500284,-0.364476539282301,
6.71545679063422));
#23895=CARTESIAN_POINT('Ctrl Pts',(-2.62820470947744,-0.416974338825206,
6.65480120525638));
#23896=CARTESIAN_POINT('Ctrl Pts',(-2.62025881842666,-0.49103185365595,
6.5068187924603));
#23897=CARTESIAN_POINT('Ctrl Pts',(-2.60833998185048,-0.482239426385862,
6.25866269895458));
#23898=CARTESIAN_POINT('Ctrl Pts',(-2.5964211452743,-0.355712410127426,
6.04504427179708));
#23899=CARTESIAN_POINT('Ctrl Pts',(-2.58450230869812,-0.142350457376832,
5.91805970308301));
#23900=CARTESIAN_POINT('Ctrl Pts',(-2.57258347212194,0.105763715802992,
5.90873487705734));
#23901=CARTESIAN_POINT('Ctrl Pts',(-2.56066463554576,0.3280581722875,6.01933440873442));
#23902=CARTESIAN_POINT('Ctrl Pts',(-2.54874579896958,0.470267002721677,
6.2228641802457));
#23903=CARTESIAN_POINT('Ctrl Pts',(-2.5368269623934,0.497673618270107,6.46963572225713));
#23904=CARTESIAN_POINT('Ctrl Pts',(-2.52490812581722,0.403587675455974,
6.69940809491329));
#23905=CARTESIAN_POINT('Ctrl Pts',(-2.51298928924104,0.210977447150787,
6.85608846546662));
#23906=CARTESIAN_POINT('Ctrl Pts',(-2.50107045266486,-0.0331368094863519,
6.90142811078917));
#23907=CARTESIAN_POINT('Ctrl Pts',(-2.48915161608868,-0.26916167858913,
6.82435854832202));
#23908=CARTESIAN_POINT('Ctrl Pts',(-2.4772327795125,-0.43947850632998,6.64369413811513));
#23909=CARTESIAN_POINT('Ctrl Pts',(-2.46531394293632,-0.502509369604788,
6.40353884455383));
#23910=CARTESIAN_POINT('Ctrl Pts',(-2.45339510636014,-0.442867104348346,
6.16251964825382));
#23911=CARTESIAN_POINT('Ctrl Pts',(-2.44147626978397,-0.275111645408374,
5.97947440914605));
#23912=CARTESIAN_POINT('Ctrl Pts',(-2.42955743320778,-0.0401956354858822,
5.89908833051357));
#23913=CARTESIAN_POINT('Ctrl Pts',(-2.41763859663161,0.204532976154487,
5.94098534715318));
#23914=CARTESIAN_POINT('Ctrl Pts',(-2.40571976005543,0.399330777640657,
6.09493751484654));
#23915=CARTESIAN_POINT('Ctrl Pts',(-2.39380092347925,0.496643520062223,
6.32336186452993));
#23916=CARTESIAN_POINT('Ctrl Pts',(-2.38188208690307,0.472715112066199,
6.57049519833277));
#23917=CARTESIAN_POINT('Ctrl Pts',(-2.36996325032689,0.333386982346306,
6.77600706087547));
#23918=CARTESIAN_POINT('Ctrl Pts',(-2.35804441375071,0.112672063828671,
6.88972767520587));
#23919=CARTESIAN_POINT('Ctrl Pts',(-2.34612557717453,-0.135548480129038,
6.88389544259157));
#23920=CARTESIAN_POINT('Ctrl Pts',(-2.33420674059835,-0.350678783287223,
6.7599341339502));
#23921=CARTESIAN_POINT('Ctrl Pts',(-2.32228790402217,-0.480201004602356,
6.54810531728136));
#23922=CARTESIAN_POINT('Ctrl Pts',(-2.31036906744599,-0.492496040045916,
6.30012087125837));
#23923=CARTESIAN_POINT('Ctrl Pts',(-2.29845023086981,-0.384562412373419,
6.07651902551736));
#23924=CARTESIAN_POINT('Ctrl Pts',(-2.28653139429363,-0.182748994814887,
5.9318857034506));
#23925=CARTESIAN_POINT('Ctrl Pts',(-2.27461255771745,0.0636773038537012,
5.90152894670173));
#23926=CARTESIAN_POINT('Ctrl Pts',(-2.26269372114127,0.294558630839998,
5.99285948055119));
#23927=CARTESIAN_POINT('Ctrl Pts',(-2.25077488456509,0.453531987451089,
6.18358159431314));
#23928=CARTESIAN_POINT('Ctrl Pts',(-2.23885604798891,0.501788628475886,
6.42713600578558));
#23929=CARTESIAN_POINT('Ctrl Pts',(-2.22693721141274,0.427548087273624,
6.6640659384009));
#23930=CARTESIAN_POINT('Ctrl Pts',(-2.21501837483655,0.24893405220493,6.83653182711616));
#23931=CARTESIAN_POINT('Ctrl Pts',(-2.20309953826038,0.00954995736342605,
6.90243105980056));
#23932=CARTESIAN_POINT('Ctrl Pts',(-2.1911807016842,-0.232165459400577,
6.84567636076067));
#23933=CARTESIAN_POINT('Ctrl Pts',(-2.17926186510802,-0.417204446142715,
6.68012249865921));
#23934=CARTESIAN_POINT('Ctrl Pts',(-2.16734302853184,-0.500394924062124,
6.44618519743075));
#23935=CARTESIAN_POINT('Ctrl Pts',(-2.15542419195566,-0.461428696189393,
6.20097232576562));
#23936=CARTESIAN_POINT('Ctrl Pts',(-2.14350535537948,-0.309817494450599,
6.00434800046925));
#23937=CARTESIAN_POINT('Ctrl Pts',(-2.1315865188033,-0.0825744709686401,
5.90430699091869));
#23938=CARTESIAN_POINT('Ctrl Pts',(-2.11966768222712,0.164828873860662,
5.92528289472092));
#23939=CARTESIAN_POINT('Ctrl Pts',(-2.10774884565094,0.371987775209309,
6.06212991827835));
#23940=CARTESIAN_POINT('Ctrl Pts',(-2.09583000907476,0.488342791333856,
6.2814932327682));
#23941=CARTESIAN_POINT('Ctrl Pts',(-2.08788411802398,0.486400997116553,
6.44696087140208));
#23942=CARTESIAN_POINT('Ctrl Pts',(-2.08391117249858,0.465688569540057,
6.52445999616013));
#23943=CARTESIAN_POINT('Ctrl Pts',(-2.64826648250425,-0.385547169725563,
6.73369355690005));
#23944=CARTESIAN_POINT('Ctrl Pts',(-2.64429353697886,-0.44107990187464,
6.66953143190698));
#23945=CARTESIAN_POINT('Ctrl Pts',(-2.63634764592807,-0.519418730749953,
6.5129940576907));
#23946=CARTESIAN_POINT('Ctrl Pts',(-2.62442880935189,-0.510118007428568,
6.25049189585148));
#23947=CARTESIAN_POINT('Ctrl Pts',(-2.61250997277571,-0.376276380452198,
6.02452404575617));
#23948=CARTESIAN_POINT('Ctrl Pts',(-2.60059113619954,-0.150579831719341,
5.89019841491327));
#23949=CARTESIAN_POINT('Ctrl Pts',(-2.58867229962336,0.111877986352145,
5.88033451451117));
#23950=CARTESIAN_POINT('Ctrl Pts',(-2.57675346304718,0.347023432783479,
5.99732787846002));
#23951=CARTESIAN_POINT('Ctrl Pts',(-2.564834626471,0.497453450012689,6.21262384103579));
#23952=CARTESIAN_POINT('Ctrl Pts',(-2.55291578989482,0.526444460181026,
6.47366140954065));
#23953=CARTESIAN_POINT('Ctrl Pts',(-2.54099695331864,0.426919346618493,
6.7167170754366));
#23954=CARTESIAN_POINT('Ctrl Pts',(-2.52907811674246,0.223174193283009,
6.88245524211623));
#23955=CARTESIAN_POINT('Ctrl Pts',(-2.51715928016628,-0.0350524704178637,
6.93041600240246));
#23956=CARTESIAN_POINT('Ctrl Pts',(-2.5052404435901,-0.284722093726431,
6.84889099741939));
#23957=CARTESIAN_POINT('Ctrl Pts',(-2.49332160701392,-0.464885050226796,
6.6577822578485));
#23958=CARTESIAN_POINT('Ctrl Pts',(-2.48140277043774,-0.531559769507257,
6.40374342750432));
#23959=CARTESIAN_POINT('Ctrl Pts',(-2.46948393386156,-0.468469545343797,
6.14879075163119));
#23960=CARTESIAN_POINT('Ctrl Pts',(-2.45756509728538,-0.291016032073294,
5.95516354586177));
#23961=CARTESIAN_POINT('Ctrl Pts',(-2.4456462607092,-0.0425193718295788,
5.87013029471448));
#23962=CARTESIAN_POINT('Ctrl Pts',(-2.43372742413302,0.216357163144678,
5.91444940567057));
#23963=CARTESIAN_POINT('Ctrl Pts',(-2.42180858755684,0.422416354717456,
6.07730165027367));
#23964=CARTESIAN_POINT('Ctrl Pts',(-2.40988975098066,0.525354811312622,
6.31893136309484));
#23965=CARTESIAN_POINT('Ctrl Pts',(-2.39797091440449,0.500043086181913,
6.58035163881449));
#23966=CARTESIAN_POINT('Ctrl Pts',(-2.38605207782831,0.352660304885654,
6.79774427841866));
#23967=CARTESIAN_POINT('Ctrl Pts',(-2.37413324125213,0.11918571055855,6.91803915687878));
#23968=CARTESIAN_POINT('Ctrl Pts',(-2.36221440467595,-0.143384627656033,
6.91186975902934));
#23969=CARTESIAN_POINT('Ctrl Pts',(-2.35029556809977,-0.370951756306248,
6.78074216492885));
#23970=CARTESIAN_POINT('Ctrl Pts',(-2.33837673152359,-0.507961743129952,
6.55666738389136));
#23971=CARTESIAN_POINT('Ctrl Pts',(-2.32645789494741,-0.520967562726117,
6.29434679258967));
#23972=CARTESIAN_POINT('Ctrl Pts',(-2.31453905837123,-0.406794220460285,
6.05781837586191));
#23973=CARTESIAN_POINT('Ctrl Pts',(-2.30262022179505,-0.193313835397505,
5.904823705531));
#23974=CARTESIAN_POINT('Ctrl Pts',(-2.29070138521887,0.067358531017915,
5.872712004543));
#23975=CARTESIAN_POINT('Ctrl Pts',(-2.27878254864269,0.311587260629241,
5.96932241712133));
#23976=CARTESIAN_POINT('Ctrl Pts',(-2.26686371206651,0.479750972411266,
6.17107030275971));
#23977=CARTESIAN_POINT('Ctrl Pts',(-2.25494487549033,0.530797361855725,
6.42870475627563));
#23978=CARTESIAN_POINT('Ctrl Pts',(-2.24302603891415,0.45226492573298,6.67933176541862));
#23979=CARTESIAN_POINT('Ctrl Pts',(-2.23110720233797,0.263325094846747,
6.86176802153349));
#23980=CARTESIAN_POINT('Ctrl Pts',(-2.2191883657618,0.0101020467317839,
6.93147693256131));
#23981=CARTESIAN_POINT('Ctrl Pts',(-2.20726952918561,-0.245587098572064,
6.87144120673232));
#23982=CARTESIAN_POINT('Ctrl Pts',(-2.19535069260943,-0.441323311848774,
6.69631656607358));
#23983=CARTESIAN_POINT('Ctrl Pts',(-2.18343185603326,-0.529323086465549,
6.44885519432254));
#23984=CARTESIAN_POINT('Ctrl Pts',(-2.17151301945708,-0.488104195118536,
6.18946640393034));
#23985=CARTESIAN_POINT('Ctrl Pts',(-2.1595941828809,-0.327728249264285,
5.98147509599461));
#23986=CARTESIAN_POINT('Ctrl Pts',(-2.14767534630472,-0.0873481558956701,
5.87565064933844));
#23987=CARTESIAN_POINT('Ctrl Pts',(-2.13575650972854,0.174357740366956,
5.89783918404992));
#23988=CARTESIAN_POINT('Ctrl Pts',(-2.12383767315236,0.393492635182685,
6.04259742479108));
#23989=CARTESIAN_POINT('Ctrl Pts',(-2.11191883657618,0.516574211951732,
6.27464227796523));
#23990=CARTESIAN_POINT('Ctrl Pts',(-2.10397294552539,0.514520161323001,
6.44967571052055));
#23991=CARTESIAN_POINT('Ctrl Pts',(-2.1,0.492610334572592,6.53165511107541));
#23992=CARTESIAN_POINT('Ctrl Pts',(-2.1,0.492610334572592,6.53165511107541));
#23993=CARTESIAN_POINT('Ctrl Pts',(-2.1,0.49635409029725,6.51110955003273));
#23994=CARTESIAN_POINT('Ctrl Pts',(-2.1,0.498800810154946,6.4903688790591));
#23995=CARTESIAN_POINT('Ctrl Pts',(-2.1,0.499959864786037,6.46955396620066));
#23996=CARTESIAN_POINT('Ctrl Pts',(-2.1,0.500651891757826,6.45712618175713));
#23997=CARTESIAN_POINT('Ctrl Pts',(-2.1,0.500884496511186,6.4446719156573));
#23998=CARTESIAN_POINT('Ctrl Pts',(-2.1,0.500656300483376,6.43221745273261));
#23999=CARTESIAN_POINT('Ctrl Pts',(-2.1,0.50051140625946,6.42430942840331));
#24000=CARTESIAN_POINT('Ctrl Pts',(-2.1,0.500180531457043,6.41639915136081));
#24001=CARTESIAN_POINT('Ctrl Pts',(-2.1,0.499663295188048,6.40850057461429));
#24002=CARTESIAN_POINT('Ctrl Pts',(-2.1,0.498282684765909,6.38741764205526));
#24003=CARTESIAN_POINT('Ctrl Pts',(-2.1,0.495579671230594,6.36646338372735));
#24004=CARTESIAN_POINT('Ctrl Pts',(-2.1,0.491553183641479,6.34576661740274));
#24005=CARTESIAN_POINT('Ctrl Pts',(-2.1,0.489189370076283,6.33361625162834));
#24006=CARTESIAN_POINT('Ctrl Pts',(-2.1,0.486369014762183,6.32155472699449));
#24007=CARTESIAN_POINT('Ctrl Pts',(-2.1,0.483088515935984,6.30960963623735));
#24008=CARTESIAN_POINT('Ctrl Pts',(-2.1,0.481387749157045,6.30341673247256));
#24009=CARTESIAN_POINT('Ctrl Pts',(-2.1,0.479562349371169,6.29725234131795));
#24010=CARTESIAN_POINT('Ctrl Pts',(-2.1,0.477614701955683,6.29113018362027));
#24011=CARTESIAN_POINT('Ctrl Pts',(-2.1,0.47691994455268,6.28894631073394));
#24012=CARTESIAN_POINT('Ctrl Pts',(-2.1,0.476209763711948,6.28676817605457));
#24013=CARTESIAN_POINT('Ctrl Pts',(-2.1,0.475484170198335,6.28459593876059));
#24014=CARTESIAN_POINT('Ctrl Pts',(-2.1,0.467396057947338,6.26038224508792));
#24015=CARTESIAN_POINT('Ctrl Pts',(-2.1,0.457396800695749,6.23689933548638));
#24016=CARTESIAN_POINT('Ctrl Pts',(-2.1,0.445625784567883,6.21434556134776));
#24017=CARTESIAN_POINT('Ctrl Pts',(-2.1,0.433955482728322,6.19198476012551));
#24018=CARTESIAN_POINT('Ctrl Pts',(-2.1,0.420542677238036,6.17053620507075));
#24019=CARTESIAN_POINT('Ctrl Pts',(-2.1,0.405485055004202,6.15022640072986));
#24020=CARTESIAN_POINT('Ctrl Pts',(-2.1,0.401547018955012,6.14491475587622));
#24021=CARTESIAN_POINT('Ctrl Pts',(-2.1,0.397496316871279,6.13968122438761));
#24022=CARTESIAN_POINT('Ctrl Pts',(-2.1,0.393334380355557,6.13453037462292));
#24023=CARTESIAN_POINT('Ctrl Pts',(-2.1,0.390073732726515,6.1304949680257));
#24024=CARTESIAN_POINT('Ctrl Pts',(-2.1,0.386745496616124,6.12651133724348));
#24025=CARTESIAN_POINT('Ctrl Pts',(-2.1,0.383357029508834,6.12258887921439));
#24026=CARTESIAN_POINT('Ctrl Pts',(-2.1,0.371904123413349,6.109331101568));
#24027=CARTESIAN_POINT('Ctrl Pts',(-2.1,0.35974458511925,6.09674730862358));
#24028=CARTESIAN_POINT('Ctrl Pts',(-2.1,0.346917810301558,6.08490712758635));
#24029=CARTESIAN_POINT('Ctrl Pts',(-2.1,0.328748103732818,6.06813497572237));
#24030=CARTESIAN_POINT('Ctrl Pts',(-2.1,0.309239814555027,6.0528527033034));
#24031=CARTESIAN_POINT('Ctrl Pts',(-2.1,0.288595198791424,6.03919240881688));
#24032=CARTESIAN_POINT('Ctrl Pts',(-2.1,0.278215530931981,6.03232430716481));
#24033=CARTESIAN_POINT('Ctrl Pts',(-2.1,0.26754829677856,6.02586696377693));
#24034=CARTESIAN_POINT('Ctrl Pts',(-2.1,0.256618135875702,6.01984205852923));
#24035=CARTESIAN_POINT('Ctrl Pts',(-2.1,0.251611498381037,6.01708230807514));
#24036=CARTESIAN_POINT('Ctrl Pts',(-2.1,0.246550009240434,6.01441370455151));
#24037=CARTESIAN_POINT('Ctrl Pts',(-2.1,0.241448312426713,6.01184414666615));
#24038=CARTESIAN_POINT('Ctrl Pts',(-2.1,0.219923137629529,6.00100261988527));
#24039=CARTESIAN_POINT('Ctrl Pts',(-2.1,0.197628752691819,5.99188954333672));
#24040=CARTESIAN_POINT('Ctrl Pts',(-2.1,0.174757433630984,5.98462368929255));
#24041=CARTESIAN_POINT('Ctrl Pts',(-2.1,0.165576347867032,5.98170700447212));
#24042=CARTESIAN_POINT('Ctrl Pts',(-2.1,0.156302149790289,5.97908854410605));
#24043=CARTESIAN_POINT('Ctrl Pts',(-2.1,0.146946980180942,5.97677835925102));
#24044=CARTESIAN_POINT('Ctrl Pts',(-2.1,0.136233092918806,5.97413264985985));
#24045=CARTESIAN_POINT('Ctrl Pts',(-2.1,0.125412970644963,5.971891235028));
#24046=CARTESIAN_POINT('Ctrl Pts',(-2.1,0.11450999527259,5.97005741415271));
#24047=CARTESIAN_POINT('Ctrl Pts',(-2.1,0.107187489851071,5.96882580875667));
#24048=CARTESIAN_POINT('Ctrl Pts',(-2.1,0.0998276196797078,5.96777809712117));
#24049=CARTESIAN_POINT('Ctrl Pts',(-2.1,0.0924376450671474,5.96691584094867));
#24050=CARTESIAN_POINT('Ctrl Pts',(-2.1,0.0866290251654119,5.96623809594594));
#24051=CARTESIAN_POINT('Ctrl Pts',(-2.1,0.0808012215405976,5.96567507726491));
#24052=CARTESIAN_POINT('Ctrl Pts',(-2.1,0.0749735051801638,5.96522838192892));
#24053=CARTESIAN_POINT('Ctrl Pts',(-2.1,0.0505591545770249,5.96335701828132));
#24054=CARTESIAN_POINT('Ctrl Pts',(-2.1,0.0260794227869884,5.96351369057634));
#24055=CARTESIAN_POINT('Ctrl Pts',(-2.1,0.00179128476957419,5.96570484843602));
#24056=CARTESIAN_POINT('Ctrl Pts',(-2.1,-0.0210365858903797,5.96776426806632));
#24057=CARTESIAN_POINT('Ctrl Pts',(-2.1,-0.0436964113942735,5.97162157501662));
#24058=CARTESIAN_POINT('Ctrl Pts',(-2.1,-0.065956881641688,5.97732901798388));
#24059=CARTESIAN_POINT('Ctrl Pts',(-2.1,-0.0673808531784219,5.97769411522767));
#24060=CARTESIAN_POINT('Ctrl Pts',(-2.1,-0.0688031806876158,5.97806679811498));
#24061=CARTESIAN_POINT('Ctrl Pts',(-2.1,-0.0702237992588386,5.97844708639908));
#24062=CARTESIAN_POINT('Ctrl Pts',(-2.1,-0.0736400801676868,5.97936159760649));
#24063=CARTESIAN_POINT('Ctrl Pts',(-2.1,-0.0770464797446285,5.9803200895664));
#24064=CARTESIAN_POINT('Ctrl Pts',(-2.1,-0.0804421690761142,5.98132232055468));
#24065=CARTESIAN_POINT('Ctrl Pts',(-2.6,-0.322335278395778,6.67898325810255));
#24066=CARTESIAN_POINT('Ctrl Pts',(-2.6,-0.339120601259259,6.66300806279478));
#24067=CARTESIAN_POINT('Ctrl Pts',(-2.6,-0.354506984127668,6.64569922647684));
#24068=CARTESIAN_POINT('Ctrl Pts',(-2.6,-0.368421126683117,6.62729272970921));
#24069=CARTESIAN_POINT('Ctrl Pts',(-2.6,-0.38257126416386,6.60857404411556));
#24070=CARTESIAN_POINT('Ctrl Pts',(-2.6,-0.395199756274692,6.58871918836577));
#24071=CARTESIAN_POINT('Ctrl Pts',(-2.6,-0.406199318727697,6.56793181289168));
#24072=CARTESIAN_POINT('Ctrl Pts',(-2.6,-0.409616043928294,6.56147476062801));
#24073=CARTESIAN_POINT('Ctrl Pts',(-2.6,-0.412875324168305,6.55492747138162));
#24074=CARTESIAN_POINT('Ctrl Pts',(-2.6,-0.415973133660165,6.54829542707107));
#24075=CARTESIAN_POINT('Ctrl Pts',(-2.6,-0.418485108810516,6.54291758490618));
#24076=CARTESIAN_POINT('Ctrl Pts',(-2.6,-0.420891069789125,6.53748311927057));
#24077=CARTESIAN_POINT('Ctrl Pts',(-2.6,-0.423182724471203,6.53201048034897));
#24078=CARTESIAN_POINT('Ctrl Pts',(-2.6,-0.42826857782987,6.51986509070635));
#24079=CARTESIAN_POINT('Ctrl Pts',(-2.6,-0.432799982024353,6.50751484134792));
#24080=CARTESIAN_POINT('Ctrl Pts',(-2.6,-0.436762141475896,6.49499689828687));
#24081=CARTESIAN_POINT('Ctrl Pts',(-2.6,-0.444013330815057,6.47208768012373));
#24082=CARTESIAN_POINT('Ctrl Pts',(-2.6,-0.449360985234842,6.44861814961569));
#24083=CARTESIAN_POINT('Ctrl Pts',(-2.6,-0.452831510630463,6.42482689824574));
#24084=CARTESIAN_POINT('Ctrl Pts',(-2.6,-0.45503518273379,6.40972021814094));
#24085=CARTESIAN_POINT('Ctrl Pts',(-2.6,-0.456481100414613,6.39448317547527));
#24086=CARTESIAN_POINT('Ctrl Pts',(-2.6,-0.457165780866727,6.37917321940029));
#24087=CARTESIAN_POINT('Ctrl Pts',(-2.6,-0.457426442969031,6.37334462399588));
#24088=CARTESIAN_POINT('Ctrl Pts',(-2.6,-0.457576507352781,6.36750526353339));
#24089=CARTESIAN_POINT('Ctrl Pts',(-2.6,-0.457615909648183,6.36167325953747));
#24090=CARTESIAN_POINT('Ctrl Pts',(-2.6,-0.457783624314556,6.33684951273631));
#24091=CARTESIAN_POINT('Ctrl Pts',(-2.6,-0.455954126792007,6.3120946330561));
#24092=CARTESIAN_POINT('Ctrl Pts',(-2.6,-0.452154218947823,6.28765697027383));
#24093=CARTESIAN_POINT('Ctrl Pts',(-2.6,-0.45115674289519,6.28124208222728));
#24094=CARTESIAN_POINT('Ctrl Pts',(-2.6,-0.450023226879442,6.27484896612481));
#24095=CARTESIAN_POINT('Ctrl Pts',(-2.6,-0.448753579228988,6.26848198366457));
#24096=CARTESIAN_POINT('Ctrl Pts',(-2.6,-0.444848441945282,6.24889864447494));
#24097=CARTESIAN_POINT('Ctrl Pts',(-2.6,-0.43965712635916,6.22956230418047));
#24098=CARTESIAN_POINT('Ctrl Pts',(-2.6,-0.433239797159997,6.21057739588651));
#24099=CARTESIAN_POINT('Ctrl Pts',(-2.6,-0.431489703713964,6.20539995172748));
#24100=CARTESIAN_POINT('Ctrl Pts',(-2.6,-0.429647959283524,6.200247760375));
#24101=CARTESIAN_POINT('Ctrl Pts',(-2.6,-0.427716565518185,6.19512580861043));
#24102=CARTESIAN_POINT('Ctrl Pts',(-2.6,-0.418824441384019,6.17154437652905));
#24103=CARTESIAN_POINT('Ctrl Pts',(-2.6,-0.408091715271334,6.14874908227563));
#24104=CARTESIAN_POINT('Ctrl Pts',(-2.6,-0.395672419048227,6.12693682894624));
#24105=CARTESIAN_POINT('Ctrl Pts',(-2.6,-0.383092367331082,6.10484223759245));
#24106=CARTESIAN_POINT('Ctrl Pts',(-2.6,-0.368781416403301,6.08375495651898));
#24107=CARTESIAN_POINT('Ctrl Pts',(-2.6,-0.352848584276632,6.06389024080292));
#24108=CARTESIAN_POINT('Ctrl Pts',(-2.6,-0.350477674538742,6.06093424104361));
#24109=CARTESIAN_POINT('Ctrl Pts',(-2.6,-0.348070766049518,6.05800535381594));
#24110=CARTESIAN_POINT('Ctrl Pts',(-2.6,-0.345628131270321,6.05510433731261));
#24111=CARTESIAN_POINT('Ctrl Pts',(-2.6,-0.341175445450433,6.04981606615654));
#24112=CARTESIAN_POINT('Ctrl Pts',(-2.6,-0.336604054215743,6.04462039757467));
#24113=CARTESIAN_POINT('Ctrl Pts',(-2.6,-0.331917615661801,6.03951989728949));
#24114=CARTESIAN_POINT('Ctrl Pts',(-2.6,-0.327197865992937,6.03438314274658));
#24115=CARTESIAN_POINT('Ctrl Pts',(-2.6,-0.322366287452079,6.02934835553984));
#24116=CARTESIAN_POINT('Ctrl Pts',(-2.6,-0.317432494385971,6.02442266645077));
#24117=CARTESIAN_POINT('Ctrl Pts',(-2.6,-0.305161639297739,6.01217196679398));
#24118=CARTESIAN_POINT('Ctrl Pts',(-2.6,-0.292249931632248,6.00058562939064));
#24119=CARTESIAN_POINT('Ctrl Pts',(-2.6,-0.278765100808516,5.98969663827542));
#24120=CARTESIAN_POINT('Ctrl Pts',(-2.6,-0.268765025516792,5.98162158472625));
#24121=CARTESIAN_POINT('Ctrl Pts',(-2.6,-0.258449546075054,5.97393011620472));
#24122=CARTESIAN_POINT('Ctrl Pts',(-2.6,-0.247843342520938,5.96663792616377));
#24123=CARTESIAN_POINT('Ctrl Pts',(-2.6,-0.241099106168833,5.96200099336216));
#24124=CARTESIAN_POINT('Ctrl Pts',(-2.6,-0.234236247932732,5.9575251822992));
#24125=CARTESIAN_POINT('Ctrl Pts',(-2.6,-0.227275760973999,5.95322352477529));
#24126=CARTESIAN_POINT('Ctrl Pts',(-2.6,-0.204751973270828,5.93930357615464));
#24127=CARTESIAN_POINT('Ctrl Pts',(-2.6,-0.181175137781382,5.92718033261133));
#24128=CARTESIAN_POINT('Ctrl Pts',(-2.6,-0.156760783265524,5.91698457674055));
#24129=CARTESIAN_POINT('Ctrl Pts',(-2.6,-0.152585729857118,5.91524101947092));
#24130=CARTESIAN_POINT('Ctrl Pts',(-2.6,-0.148386104006604,5.91355392287942));
#24131=CARTESIAN_POINT('Ctrl Pts',(-2.6,-0.144162892324896,5.91192406382743));
#24132=CARTESIAN_POINT('Ctrl Pts',(-2.6,-0.140229927621667,5.91040621944599));
#24133=CARTESIAN_POINT('Ctrl Pts',(-2.6,-0.136276507298105,5.90893801577657));
#24134=CARTESIAN_POINT('Ctrl Pts',(-2.6,-0.132303594671778,5.90751949357016));
#24135=CARTESIAN_POINT('Ctrl Pts',(-2.3579681670589,0.426284649716722,6.39998978457651));
#24136=CARTESIAN_POINT('Ctrl Pts',(-2.35918653419807,0.426303967962151,
6.37823165906101));
#24137=CARTESIAN_POINT('Ctrl Pts',(-2.36040490133724,0.424667502862756,
6.35647641245579));
#24138=CARTESIAN_POINT('Ctrl Pts',(-2.36162326847641,0.421350422927922,
6.33498050516036));
#24139=CARTESIAN_POINT('Ctrl Pts',(-2.3655962140018,0.41053383286997,6.26488499293085));
#24140=CARTESIAN_POINT('Ctrl Pts',(-2.3695691595272,0.381846728178515,6.19754711846157));
#24141=CARTESIAN_POINT('Ctrl Pts',(-2.37354210505259,0.338790672280628,
6.14118617891461));
#24142=CARTESIAN_POINT('Ctrl Pts',(-2.37751505057798,0.295734616382741,
6.08482523936765));
#24143=CARTESIAN_POINT('Ctrl Pts',(-2.38148799610338,0.238309609278423,
6.03944123474302));
#24144=CARTESIAN_POINT('Ctrl Pts',(-2.38546094162877,0.173524978230831,
6.01057376109627));
#24145=CARTESIAN_POINT('Ctrl Pts',(-2.38943388715416,0.10874034718324,5.98170628744951));
#24146=CARTESIAN_POINT('Ctrl Pts',(-2.39340683267956,0.036596092192376,
5.96935534478063));
#24147=CARTESIAN_POINT('Ctrl Pts',(-2.39737977820495,-0.0341018201830637,
5.97502849571334));
#24148=CARTESIAN_POINT('Ctrl Pts',(-2.40135272373034,-0.104799732558504,
5.98070164664604));
#24149=CARTESIAN_POINT('Ctrl Pts',(-2.40532566925574,-0.174051302318518,
6.00439889118032));
#24150=CARTESIAN_POINT('Ctrl Pts',(-2.40929861478113,-0.233403645578344,
6.0432277310782));
#24151=CARTESIAN_POINT('Ctrl Pts',(-2.41327156030652,-0.29275598883817,
6.08205657097609));
#24152=CARTESIAN_POINT('Ctrl Pts',(-2.41724450583192,-0.342209105597808,
6.13601700623758));
#24153=CARTESIAN_POINT('Ctrl Pts',(-2.42121745135731,-0.375726721884694,
6.19852259672729));
#24154=CARTESIAN_POINT('Ctrl Pts',(-2.4251903968827,-0.40924433817158,6.261028187217));
#24155=CARTESIAN_POINT('Ctrl Pts',(-2.4291633424081,-0.426826453985716,
6.33207893293493));
#24156=CARTESIAN_POINT('Ctrl Pts',(-2.43313628793349,-0.426326986682199,
6.40300234245982));
#24157=CARTESIAN_POINT('Ctrl Pts',(-2.43710923345888,-0.425827519378683,
6.4739257519847));
#24158=CARTESIAN_POINT('Ctrl Pts',(-2.44108217898427,-0.407246468957515,
6.54472182531654));
#24159=CARTESIAN_POINT('Ctrl Pts',(-2.44505512450967,-0.372851848709961,
6.60674915389561));
#24160=CARTESIAN_POINT('Ctrl Pts',(-2.44902807003506,-0.338457228462407,
6.66877648247468));
#24161=CARTESIAN_POINT('Ctrl Pts',(-2.45300101556045,-0.288249038388467,
6.72203506630097));
#24162=CARTESIAN_POINT('Ctrl Pts',(-2.45697396108585,-0.228355716569631,
6.76002413778667));
#24163=CARTESIAN_POINT('Ctrl Pts',(-2.46094690661124,-0.168462394750795,
6.79801320927237));
#24164=CARTESIAN_POINT('Ctrl Pts',(-2.46491985213663,-0.0988839411870617,
6.82073276841748));
#24165=CARTESIAN_POINT('Ctrl Pts',(-2.46889279766203,-0.0281131406535831,
6.82540964542417));
#24166=CARTESIAN_POINT('Ctrl Pts',(-2.47286574318742,0.0426576598798955,
6.83008652243086));
#24167=CARTESIAN_POINT('Ctrl Pts',(-2.47683868871281,0.11462080738312,6.81672071729912));
#24168=CARTESIAN_POINT('Ctrl Pts',(-2.48081163423821,0.178992444175497,
6.78694368501647));
#24169=CARTESIAN_POINT('Ctrl Pts',(-2.4847845797636,0.243364080967874,6.75716665273382));
#24170=CARTESIAN_POINT('Ctrl Pts',(-2.48875752528899,0.300144207049405,
6.71097839330025));
#24171=CARTESIAN_POINT('Ctrl Pts',(-2.49273047081439,0.342402203643058,
6.65401663255403));
#24172=CARTESIAN_POINT('Ctrl Pts',(-2.49670341633978,0.384660200236712,
6.59705487180782));
#24173=CARTESIAN_POINT('Ctrl Pts',(-2.50067636186517,0.41239606734249,6.52931960974896));
#24174=CARTESIAN_POINT('Ctrl Pts',(-2.50464930739057,0.422224363177276,
6.45907873054876));
#24175=CARTESIAN_POINT('Ctrl Pts',(-2.50575559394668,0.424961101318294,
6.4395198063571));
#24176=CARTESIAN_POINT('Ctrl Pts',(-2.50686188050279,0.426309336731809,
6.41976660365709));
#24177=CARTESIAN_POINT('Ctrl Pts',(-2.50796816705891,0.426290360635438,
6.40001083203199));
#24178=CARTESIAN_POINT('Ctrl Pts',(-2.6,0.132288496556895,5.90755938055567));
#24179=CARTESIAN_POINT('Ctrl Pts',(-2.59602705447461,0.214239653399634,
5.92957461427473));
#24180=CARTESIAN_POINT('Ctrl Pts',(-2.58808116342382,0.366850103542102,
6.0153123398751));
#24181=CARTESIAN_POINT('Ctrl Pts',(-2.57616232684764,0.506266020658281,
6.23792666630748));
#24182=CARTESIAN_POINT('Ctrl Pts',(-2.56424349027146,0.522062886964902,
6.50008215105946));
#24183=CARTESIAN_POINT('Ctrl Pts',(-2.55232465369528,0.410425773087965,
6.73782039475945));
#24184=CARTESIAN_POINT('Ctrl Pts',(-2.54040581711911,0.19858907062663,6.89308342832313));
#24185=CARTESIAN_POINT('Ctrl Pts',(-2.52848698054292,-0.0617246536500735,
6.92797742227401));
#24186=CARTESIAN_POINT('Ctrl Pts',(-2.51656814396674,-0.306971377021502,
6.8339796336226));
#24187=CARTESIAN_POINT('Ctrl Pts',(-2.50464930739056,-0.477279320739804,
6.63403891232169));
#24188=CARTESIAN_POINT('Ctrl Pts',(-2.49273047081439,-0.531073600862929,
6.3769640630774));
#24189=CARTESIAN_POINT('Ctrl Pts',(-2.48081163423821,-0.455221493256117,
6.12551290982166));
#24190=CARTESIAN_POINT('Ctrl Pts',(-2.46889279766203,-0.268240284898955,
5.94106977614238));
#24191=CARTESIAN_POINT('Ctrl Pts',(-2.45697396108585,-0.0157759417689948,
5.86866121228054));
#24192=CARTESIAN_POINT('Ctrl Pts',(-2.44505512450967,0.240539628301038,
5.92596363104932));
#24193=CARTESIAN_POINT('Ctrl Pts',(-2.43313628793349,0.438134411540293,
6.09898832463164));
#24194=CARTESIAN_POINT('Ctrl Pts',(-2.42121745135731,0.528771348081292,
6.34549630925116));
#24195=CARTESIAN_POINT('Ctrl Pts',(-2.40929861478113,0.490324055555984,
6.60530979488368));
#24196=CARTESIAN_POINT('Ctrl Pts',(-2.39737977820495,0.332178326477852,
6.81500283186379));
#24197=CARTESIAN_POINT('Ctrl Pts',(-2.38546094162877,0.092940867251264,
6.92338493135519));
#24198=CARTESIAN_POINT('Ctrl Pts',(-2.37354210505259,-0.168985416607936,
6.90399773818908));
#24199=CARTESIAN_POINT('Ctrl Pts',(-2.36162326847641,-0.38965879870384,
6.76157407502307));
#24200=CARTESIAN_POINT('Ctrl Pts',(-2.34970443190023,-0.515208255680234,
6.5308825596382));
#24201=CARTESIAN_POINT('Ctrl Pts',(-2.33778559532405,-0.514984518987432,
6.26823985300105));
#24202=CARTESIAN_POINT('Ctrl Pts',(-2.32586675874787,-0.389042207488899,
6.03776257519368));
#24203=CARTESIAN_POINT('Ctrl Pts',(-2.31394792217169,-0.168126493747137,
5.89571508724314));
#24204=CARTESIAN_POINT('Ctrl Pts',(-2.30202908559551,0.0938324405162212,
5.87677417471489));
#24205=CARTESIAN_POINT('Ctrl Pts',(-2.29011024901934,0.332884898468083,
5.98556371357228));
#24206=CARTESIAN_POINT('Ctrl Pts',(-2.27819141244316,0.490673136844557,
6.19552588451105));
#24207=CARTESIAN_POINT('Ctrl Pts',(-2.26627257586698,0.528677721240565,
6.45540449655913));
#24208=CARTESIAN_POINT('Ctrl Pts',(-2.2543537392908,0.437620931409163,6.70175770318116));
#24209=CARTESIAN_POINT('Ctrl Pts',(-2.24243490271462,0.239731649313908,
6.87444549491937));
#24210=CARTESIAN_POINT('Ctrl Pts',(-2.23051606613844,-0.0166811816108265,
6.93131114145764));
#24211=CARTESIAN_POINT('Ctrl Pts',(-2.21859722956226,-0.269021783055123,
6.85847254173578));
#24212=CARTESIAN_POINT('Ctrl Pts',(-2.20667839298608,-0.455688500581004,
6.67371112931225));
#24213=CARTESIAN_POINT('Ctrl Pts',(-2.1947595564099,-0.53111204424701,6.42213106706975));
#24214=CARTESIAN_POINT('Ctrl Pts',(-2.18284071983372,-0.476879959029563,
6.1651483330086));
#24215=CARTESIAN_POINT('Ctrl Pts',(-2.17092188325754,-0.306231393425269,
5.96549786619889));
#24216=CARTESIAN_POINT('Ctrl Pts',(-2.15900304668136,-0.0608253588918372,
5.8719184725451));
#24217=CARTESIAN_POINT('Ctrl Pts',(-2.14708421010518,0.199429574813985,
5.90725502825896));
#24218=CARTESIAN_POINT('Ctrl Pts',(-2.135165373529,0.410999230249818,6.06288076079265));
#24219=CARTESIAN_POINT('Ctrl Pts',(-2.12324653695282,0.522235994732442,
6.30080495423084));
#24220=CARTESIAN_POINT('Ctrl Pts',(-2.11132770037665,0.505982491766854,
6.56294356165447));
#24221=CARTESIAN_POINT('Ctrl Pts',(-2.09940886380046,0.366211204665212,
6.78530674521469));
#24222=CARTESIAN_POINT('Ctrl Pts',(-2.08749002722428,0.137033499838515,
6.91360287657764));
#24223=CARTESIAN_POINT('Ctrl Pts',(-2.07557119064811,-0.125581190928044,
6.91652919922544));
#24224=CARTESIAN_POINT('Ctrl Pts',(-2.06365235407193,-0.357565218298462,
6.79333282215497));
#24225=CARTESIAN_POINT('Ctrl Pts',(-2.05570646302114,-0.453961018087142,
6.64722068416873));
#24226=CARTESIAN_POINT('Ctrl Pts',(-2.05173351749575,-0.481760682217403,
6.56704686488953));
#24227=CARTESIAN_POINT('Ctrl Pts',(-2.61608882750142,0.12505876634041,5.9344718704462));
#24228=CARTESIAN_POINT('Ctrl Pts',(-2.61211588197602,0.202531190940192,
5.95528394436993));
#24229=CARTESIAN_POINT('Ctrl Pts',(-2.60416999092524,0.346801290927786,
6.03633599705392));
#24230=CARTESIAN_POINT('Ctrl Pts',(-2.59225115434906,0.478597955464431,
6.24678417477103));
#24231=CARTESIAN_POINT('Ctrl Pts',(-2.58033231777288,0.493531503458158,
6.49461253752179));
#24232=CARTESIAN_POINT('Ctrl Pts',(-2.5684134811967,0.387995496151209,6.71935809169225));
#24233=CARTESIAN_POINT('Ctrl Pts',(-2.55649464462052,0.187735931903752,
6.86613580813106));
#24234=CARTESIAN_POINT('Ctrl Pts',(-2.54457580804434,-0.0583513248632879,
6.89912280208567));
#24235=CARTESIAN_POINT('Ctrl Pts',(-2.53265697146816,-0.290195010989602,
6.81026210902899));
#24236=CARTESIAN_POINT('Ctrl Pts',(-2.52073813489198,-0.451195414605367,
6.62124839583474));
#24237=CARTESIAN_POINT('Ctrl Pts',(-2.5088192983158,-0.50204977067914,6.37822300556726));
#24238=CARTESIAN_POINT('Ctrl Pts',(-2.49690046173962,-0.430343074719011,
6.14051396933589));
#24239=CARTESIAN_POINT('Ctrl Pts',(-2.48498162516344,-0.253580621031822,
5.96615088140125));
#24240=CARTESIAN_POINT('Ctrl Pts',(-2.47306278858726,-0.0149137670080035,
5.89769953525455));
#24241=CARTESIAN_POINT('Ctrl Pts',(-2.46114395201109,0.227393839632693,
5.95187030585109));
#24242=CARTESIAN_POINT('Ctrl Pts',(-2.44922511543491,0.414189823186519,
6.11543898558529));
#24243=CARTESIAN_POINT('Ctrl Pts',(-2.43730627885873,0.499873338864062,
6.34847500347002));
#24244=CARTESIAN_POINT('Ctrl Pts',(-2.42538744228255,0.463527238503961,
6.59408936025449));
#24245=CARTESIAN_POINT('Ctrl Pts',(-2.41346860570637,0.314024369431667,
6.79232241299485));
#24246=CARTESIAN_POINT('Ctrl Pts',(-2.40154976913019,0.0878615337203718,
6.89478129648476));
#24247=CARTESIAN_POINT('Ctrl Pts',(-2.38963093255401,-0.159750154250334,
6.87645363744213));
#24248=CARTESIAN_POINT('Ctrl Pts',(-2.37771209597783,-0.368363462643409,
6.74181360390328));
#24249=CARTESIAN_POINT('Ctrl Pts',(-2.36579325940165,-0.487051486264749,
6.52372966561601));
#24250=CARTESIAN_POINT('Ctrl Pts',(-2.35387442282547,-0.486839977059375,
6.27544070825967));
#24251=CARTESIAN_POINT('Ctrl Pts',(-2.34195558624929,-0.367780568902201,
6.05755929920087));
#24252=CARTESIAN_POINT('Ctrl Pts',(-2.33003674967311,-0.158938172587915,
5.92327488243597));
#24253=CARTESIAN_POINT('Ctrl Pts',(-2.31811791309693,0.0887043814019138,
5.90536911424148));
#24254=CARTESIAN_POINT('Ctrl Pts',(-2.30619907652075,0.314692326387328,
6.0082131700313));
#24255=CARTESIAN_POINT('Ctrl Pts',(-2.29428023994457,0.463857242067669,
6.20670064822607));
#24256=CARTESIAN_POINT('Ctrl Pts',(-2.28236140336839,0.499784828846167,
6.45237657218681));
#24257=CARTESIAN_POINT('Ctrl Pts',(-2.27044256679221,0.413704405380657,
6.68526627088336));
#24258=CARTESIAN_POINT('Ctrl Pts',(-2.25852373021604,0.226630017698138,
6.84851646087657));
#24259=CARTESIAN_POINT('Ctrl Pts',(-2.24660489363986,-0.0157695343710637,
6.90227432938608));
#24260=CARTESIAN_POINT('Ctrl Pts',(-2.23468605706368,-0.254319409345632,
6.83341644937185));
#24261=CARTESIAN_POINT('Ctrl Pts',(-2.2227672204875,-0.430784559515061,
6.65875247702062));
#24262=CARTESIAN_POINT('Ctrl Pts',(-2.21084838391132,-0.502086113084658,
6.42092157683831));
#24263=CARTESIAN_POINT('Ctrl Pts',(-2.19892954733514,-0.450817878507322,
6.1779832675451));
#24264=CARTESIAN_POINT('Ctrl Pts',(-2.18701071075896,-0.289495468413598,
5.98924394607454));
#24265=CARTESIAN_POINT('Ctrl Pts',(-2.17509187418278,-0.05750117767764,
5.90077878221055));
#24266=CARTESIAN_POINT('Ctrl Pts',(-2.1631730376066,0.188530501496047,5.93418415137954));
#24267=CARTESIAN_POINT('Ctrl Pts',(-2.15125420103042,0.388537613168766,
6.08130474484033));
#24268=CARTESIAN_POINT('Ctrl Pts',(-2.13933536445424,0.493695150671756,
6.30622608636544));
#24269=CARTESIAN_POINT('Ctrl Pts',(-2.12741652787806,0.478329921778157,
6.55403849415475));
#24270=CARTESIAN_POINT('Ctrl Pts',(-2.11549769130188,0.346197308665989,
6.76424925426879));
#24271=CARTESIAN_POINT('Ctrl Pts',(-2.1035788547257,0.129544449314556,6.88553384311886));
#24272=CARTESIAN_POINT('Ctrl Pts',(-2.09166001814953,-0.11871802327322,
6.88830023860881));
#24273=CARTESIAN_POINT('Ctrl Pts',(-2.07974118157334,-0.338023836164873,
6.77183669616154));
#24274=CARTESIAN_POINT('Ctrl Pts',(-2.07179529052256,-0.429151486079503,
6.63370976752069));
#24275=CARTESIAN_POINT('Ctrl Pts',(-2.06782234499716,-0.455431864126683,
6.55791754678483));
#24276=CARTESIAN_POINT('Ctrl Pts',(-2.63217765500284,0.117829036123926,
5.96138436033673));
#24277=CARTESIAN_POINT('Ctrl Pts',(-2.62820470947744,0.190822728480749,
5.98099327446513));
#24278=CARTESIAN_POINT('Ctrl Pts',(-2.62025881842666,0.326752478313469,
6.05735965423274));
#24279=CARTESIAN_POINT('Ctrl Pts',(-2.60833998185048,0.450929890270581,
6.25564168323458));
#24280=CARTESIAN_POINT('Ctrl Pts',(-2.5964211452743,0.465000119951414,6.48914292398412));
#24281=CARTESIAN_POINT('Ctrl Pts',(-2.58450230869812,0.365565219214455,
6.70089578862506));
#24282=CARTESIAN_POINT('Ctrl Pts',(-2.57258347212194,0.176882793180874,
6.83918818793898));
#24283=CARTESIAN_POINT('Ctrl Pts',(-2.56066463554576,-0.0549779960765018,
6.87026818189733));
#24284=CARTESIAN_POINT('Ctrl Pts',(-2.54874579896958,-0.273418644957702,
6.78654458443538));
#24285=CARTESIAN_POINT('Ctrl Pts',(-2.5368269623934,-0.42511150847093,6.60845787934779));
#24286=CARTESIAN_POINT('Ctrl Pts',(-2.52490812581722,-0.473025940495352,
6.37948194805711));
#24287=CARTESIAN_POINT('Ctrl Pts',(-2.51298928924104,-0.405464656181905,
6.15551502885011));
#24288=CARTESIAN_POINT('Ctrl Pts',(-2.50107045266486,-0.23892095716469,
5.99123198666013));
#24289=CARTESIAN_POINT('Ctrl Pts',(-2.48915161608868,-0.014051592247013,
5.92673785822857));
#24290=CARTESIAN_POINT('Ctrl Pts',(-2.4772327795125,0.214248050964349,5.97777698065287));
#24291=CARTESIAN_POINT('Ctrl Pts',(-2.46531394293632,0.390245234832745,
6.13188964653893));
#24292=CARTESIAN_POINT('Ctrl Pts',(-2.45339510636014,0.470975329646833,
6.35145369768889));
#24293=CARTESIAN_POINT('Ctrl Pts',(-2.44147626978396,0.436730421451937,
6.5828689256253));
#24294=CARTESIAN_POINT('Ctrl Pts',(-2.42955743320779,0.295870412385483,
6.76964199412591));
#24295=CARTESIAN_POINT('Ctrl Pts',(-2.41763859663161,0.0827822001894799,
6.86617766161433));
#24296=CARTESIAN_POINT('Ctrl Pts',(-2.40571976005543,-0.150514891892733,
6.84890953669518));
#24297=CARTESIAN_POINT('Ctrl Pts',(-2.39380092347925,-0.347068126582978,
6.7220531327835));
#24298=CARTESIAN_POINT('Ctrl Pts',(-2.38188208690307,-0.458894716849264,
6.51657677159381));
#24299=CARTESIAN_POINT('Ctrl Pts',(-2.36996325032689,-0.458695435131318,
6.28264156351829));
#24300=CARTESIAN_POINT('Ctrl Pts',(-2.35804441375071,-0.346518930315503,
6.07735602320807));
#24301=CARTESIAN_POINT('Ctrl Pts',(-2.34612557717453,-0.149749851428694,
5.9508346776288));
#24302=CARTESIAN_POINT('Ctrl Pts',(-2.33420674059835,0.0835763222876063,
5.93396405376808));
#24303=CARTESIAN_POINT('Ctrl Pts',(-2.32228790402217,0.296499754306572,
6.03086262649031));
#24304=CARTESIAN_POINT('Ctrl Pts',(-2.31036906744599,0.437041347290782,
6.2178754119411));
#24305=CARTESIAN_POINT('Ctrl Pts',(-2.29845023086981,0.470891936451769,
6.44934864781448));
#24306=CARTESIAN_POINT('Ctrl Pts',(-2.28653139429363,0.389787879352151,
6.66877483858555));
#24307=CARTESIAN_POINT('Ctrl Pts',(-2.27461255771745,0.213528386082369,
6.82258742683378));
#24308=CARTESIAN_POINT('Ctrl Pts',(-2.26269372114127,-0.0148578871313011,
6.87323751731453));
#24309=CARTESIAN_POINT('Ctrl Pts',(-2.2507748845651,-0.239617035636141,
6.80836035700791));
#24310=CARTESIAN_POINT('Ctrl Pts',(-2.23885604798891,-0.405880618449119,
6.64379382472899));
#24311=CARTESIAN_POINT('Ctrl Pts',(-2.22693721141274,-0.473060181922306,
6.41971208660688));
#24312=CARTESIAN_POINT('Ctrl Pts',(-2.21501837483656,-0.424755797985082,
6.1908182020816));
#24313=CARTESIAN_POINT('Ctrl Pts',(-2.20309953826038,-0.272759543401928,
6.01299002595018));
#24314=CARTESIAN_POINT('Ctrl Pts',(-2.1911807016842,-0.0541769964634428,
5.92963909187599));
#24315=CARTESIAN_POINT('Ctrl Pts',(-2.17926186510802,0.17763142817811,5.96111327450012));
#24316=CARTESIAN_POINT('Ctrl Pts',(-2.16734302853184,0.366075996087714,
6.099728728888));
#24317=CARTESIAN_POINT('Ctrl Pts',(-2.15542419195566,0.465154306611069,
6.31164721850004));
#24318=CARTESIAN_POINT('Ctrl Pts',(-2.14350535537948,0.450677351789461,
6.54513342665504));
#24319=CARTESIAN_POINT('Ctrl Pts',(-2.1315865188033,0.326183412666766,6.74319176332289));
#24320=CARTESIAN_POINT('Ctrl Pts',(-2.11966768222712,0.122055398790597,
6.85746480966008));
#24321=CARTESIAN_POINT('Ctrl Pts',(-2.10774884565094,-0.111854855618396,
6.8600712779922));
#24322=CARTESIAN_POINT('Ctrl Pts',(-2.09583000907476,-0.318482454031284,
6.7503405701681));
#24323=CARTESIAN_POINT('Ctrl Pts',(-2.08788411802398,-0.404341954071864,
6.62019885087265));
#24324=CARTESIAN_POINT('Ctrl Pts',(-2.08391117249858,-0.429103046035963,
6.54878822868013));
#24325=CARTESIAN_POINT('Ctrl Pts',(-2.64826648250425,0.110599305907441,
5.98829685022726));
#24326=CARTESIAN_POINT('Ctrl Pts',(-2.64429353697886,0.179114266021306,
6.00670260456034));
#24327=CARTESIAN_POINT('Ctrl Pts',(-2.63634764592807,0.306703665699153,
6.07838331141156));
#24328=CARTESIAN_POINT('Ctrl Pts',(-2.6244288093519,0.423261825076731,6.26449919169813));
#24329=CARTESIAN_POINT('Ctrl Pts',(-2.61250997277572,0.436468736444671,
6.48367331044645));
#24330=CARTESIAN_POINT('Ctrl Pts',(-2.60059113619953,0.3431349422777,6.68243348555786));
#24331=CARTESIAN_POINT('Ctrl Pts',(-2.58867229962336,0.166029654457996,
6.81224056774691));
#24332=CARTESIAN_POINT('Ctrl Pts',(-2.57675346304718,-0.0516046672897163,
6.84141356170898));
#24333=CARTESIAN_POINT('Ctrl Pts',(-2.564834626471,-0.256642278925802,6.76282705984177));
#24334=CARTESIAN_POINT('Ctrl Pts',(-2.55291578989482,-0.399027602336494,
6.59566736286083));
#24335=CARTESIAN_POINT('Ctrl Pts',(-2.54099695331864,-0.444002110311564,
6.38074089054697));
#24336=CARTESIAN_POINT('Ctrl Pts',(-2.52907811674246,-0.380586237644799,
6.17051608836433));
#24337=CARTESIAN_POINT('Ctrl Pts',(-2.51715928016628,-0.224261293297557,
6.016313091919));
#24338=CARTESIAN_POINT('Ctrl Pts',(-2.5052404435901,-0.0131894174860218,
5.95577618120258));
#24339=CARTESIAN_POINT('Ctrl Pts',(-2.49332160701392,0.201102262296004,
6.00368365545465));
#24340=CARTESIAN_POINT('Ctrl Pts',(-2.48140277043774,0.366300646478971,
6.14834030749258));
#24341=CARTESIAN_POINT('Ctrl Pts',(-2.46948393386156,0.442077320429603,
6.35443239190776));
#24342=CARTESIAN_POINT('Ctrl Pts',(-2.45756509728538,0.409933604399914,
6.57164849099611));
#24343=CARTESIAN_POINT('Ctrl Pts',(-2.4456462607092,0.277716455339298,6.74696157525698));
#24344=CARTESIAN_POINT('Ctrl Pts',(-2.43372742413302,0.0777028666585877,
6.8375740267439));
#24345=CARTESIAN_POINT('Ctrl Pts',(-2.42180858755684,-0.141279629535131,
6.82136543594824));
#24346=CARTESIAN_POINT('Ctrl Pts',(-2.40988975098066,-0.325772790522547,
6.70229266166372));
#24347=CARTESIAN_POINT('Ctrl Pts',(-2.39797091440449,-0.430737947433779,
6.50942387757162));
#24348=CARTESIAN_POINT('Ctrl Pts',(-2.38605207782831,-0.43055089320326,
6.28984241877691));
#24349=CARTESIAN_POINT('Ctrl Pts',(-2.37413324125213,-0.325257291728805,
6.09715274721527));
#24350=CARTESIAN_POINT('Ctrl Pts',(-2.36221440467595,-0.140561530269473,
5.97839447282163));
#24351=CARTESIAN_POINT('Ctrl Pts',(-2.35029556809977,0.0784482631732989,
5.96255899329468));
#24352=CARTESIAN_POINT('Ctrl Pts',(-2.33837673152359,0.278307182225817,
6.05351208294933));
#24353=CARTESIAN_POINT('Ctrl Pts',(-2.32645789494741,0.410225452513894,
6.22905017565613));
#24354=CARTESIAN_POINT('Ctrl Pts',(-2.31453905837123,0.44199904405737,6.44632072344216));
#24355=CARTESIAN_POINT('Ctrl Pts',(-2.30262022179505,0.365871353323644,
6.65228340628776));
#24356=CARTESIAN_POINT('Ctrl Pts',(-2.29070138521887,0.200426754466599,
6.79665839279099));
#24357=CARTESIAN_POINT('Ctrl Pts',(-2.27878254864269,-0.0139462398915382,
6.84420070524297));
#24358=CARTESIAN_POINT('Ctrl Pts',(-2.26686371206651,-0.22491466192665,
6.78330426464398));
#24359=CARTESIAN_POINT('Ctrl Pts',(-2.25494487549033,-0.380976677383177,
6.62883517243736));
#24360=CARTESIAN_POINT('Ctrl Pts',(-2.24302603891415,-0.444034250759953,
6.41850259637544));
#24361=CARTESIAN_POINT('Ctrl Pts',(-2.23110720233797,-0.398693717462841,
6.2036531366181));
#24362=CARTESIAN_POINT('Ctrl Pts',(-2.2191883657618,-0.256023618390257,
6.03673610582583));
#24363=CARTESIAN_POINT('Ctrl Pts',(-2.20726952918561,-0.0508528152492455,
5.95849940154143));
#24364=CARTESIAN_POINT('Ctrl Pts',(-2.19535069260944,0.166732354860172,
5.9880423976207));
#24365=CARTESIAN_POINT('Ctrl Pts',(-2.18343185603326,0.343614379006663,
6.11815271293568));
#24366=CARTESIAN_POINT('Ctrl Pts',(-2.17151301945708,0.436613462550383,
6.31706835063465));
#24367=CARTESIAN_POINT('Ctrl Pts',(-2.1595941828809,0.423024781800764,6.53622835915532));
#24368=CARTESIAN_POINT('Ctrl Pts',(-2.14767534630472,0.306169516667542,
6.72213427237698));
#24369=CARTESIAN_POINT('Ctrl Pts',(-2.13575650972854,0.114566348266639,
6.8293957762013));
#24370=CARTESIAN_POINT('Ctrl Pts',(-2.12383767315236,-0.104991687963572,
6.83184231737557));
#24371=CARTESIAN_POINT('Ctrl Pts',(-2.11191883657618,-0.298941071897694,
6.72884444417467));
#24372=CARTESIAN_POINT('Ctrl Pts',(-2.10397294552539,-0.379532422064226,
6.60668793422461));
#24373=CARTESIAN_POINT('Ctrl Pts',(-2.1,-0.402774227945242,6.53965891057542));
#24374=CARTESIAN_POINT('Ctrl Pts',(-2.1,-0.402774227945242,6.53965891057542));
#24375=CARTESIAN_POINT('Ctrl Pts',(-2.1,-0.398484638758285,6.55741240483299));
#24376=CARTESIAN_POINT('Ctrl Pts',(-2.1,-0.393037299189535,6.57484669319261));
#24377=CARTESIAN_POINT('Ctrl Pts',(-2.1,-0.386509552509357,6.59187123411703));
#24378=CARTESIAN_POINT('Ctrl Pts',(-2.1,-0.381753507363848,6.60427512924121));
#24379=CARTESIAN_POINT('Ctrl Pts',(-2.1,-0.376423475271725,6.61646161573661));
#24380=CARTESIAN_POINT('Ctrl Pts',(-2.1,-0.370542725187782,6.62839523023791));
#24381=CARTESIAN_POINT('Ctrl Pts',(-2.1,-0.367213725298235,6.63515066122709));
#24382=CARTESIAN_POINT('Ctrl Pts',(-2.1,-0.363707525435473,6.6418256648993));
#24383=CARTESIAN_POINT('Ctrl Pts',(-2.1,-0.360036351586671,6.64839942538541));
#24384=CARTESIAN_POINT('Ctrl Pts',(-2.1,-0.35176296808893,6.66321409877431));
#24385=CARTESIAN_POINT('Ctrl Pts',(-2.1,-0.342644371178579,6.67753242868165));
#24386=CARTESIAN_POINT('Ctrl Pts',(-2.1,-0.332730966942087,6.69128302674014));
#24387=CARTESIAN_POINT('Ctrl Pts',(-2.1,-0.326097681493147,6.70048386631449));
#24388=CARTESIAN_POINT('Ctrl Pts',(-2.1,-0.319108257560132,6.70943048957354));
#24389=CARTESIAN_POINT('Ctrl Pts',(-2.1,-0.311774677324918,6.7181003705903));
#24390=CARTESIAN_POINT('Ctrl Pts',(-2.1,-0.308148267079993,6.7223875733389));
#24391=CARTESIAN_POINT('Ctrl Pts',(-2.1,-0.304437253383367,6.7266073471557));
#24392=CARTESIAN_POINT('Ctrl Pts',(-2.1,-0.30065086413981,6.73074867775903));
#24393=CARTESIAN_POINT('Ctrl Pts',(-2.1,-0.284450150446919,6.74846806873983));
#24394=CARTESIAN_POINT('Ctrl Pts',(-2.1,-0.26684239953173,6.76479115222895));
#24395=CARTESIAN_POINT('Ctrl Pts',(-2.1,-0.24806300232608,6.77963444611442));
#24396=CARTESIAN_POINT('Ctrl Pts',(-2.1,-0.229015002355758,6.79469004445943));
#24397=CARTESIAN_POINT('Ctrl Pts',(-2.1,-0.208760629118366,6.80822418203225));
#24398=CARTESIAN_POINT('Ctrl Pts',(-2.1,-0.187501868003905,6.82011881527523));
#24399=CARTESIAN_POINT('Ctrl Pts',(-2.1,-0.182121127272195,6.8231294299218));
#24400=CARTESIAN_POINT('Ctrl Pts',(-2.1,-0.176675868974013,6.82603481851803));
#24401=CARTESIAN_POINT('Ctrl Pts',(-2.1,-0.171169051786272,6.82883264150109));
#24402=CARTESIAN_POINT('Ctrl Pts',(-2.1,-0.165595855256536,6.83166418952754));
#24403=CARTESIAN_POINT('Ctrl Pts',(-2.1,-0.159966248284264,6.83438207494035));
#24404=CARTESIAN_POINT('Ctrl Pts',(-2.1,-0.154290568068188,6.83698163141168));
#24405=CARTESIAN_POINT('Ctrl Pts',(-2.1,-0.139973144289019,6.84353925097815));
#24406=CARTESIAN_POINT('Ctrl Pts',(-2.1,-0.1253500812197,6.84935087179354));
#24407=CARTESIAN_POINT('Ctrl Pts',(-2.1,-0.110478871969928,6.85439100862466));
#24408=CARTESIAN_POINT('Ctrl Pts',(-2.1,-0.091606231881728,6.86078730678786));
#24409=CARTESIAN_POINT('Ctrl Pts',(-2.1,-0.0723341026865624,6.8659419398207));
#24410=CARTESIAN_POINT('Ctrl Pts',(-2.1,-0.0527866493565085,6.86986556285165));
#24411=CARTESIAN_POINT('Ctrl Pts',(-2.1,-0.0364584381349322,6.87314301002196));
#24412=CARTESIAN_POINT('Ctrl Pts',(-2.1,-0.0199377431301133,6.87556121981262));
#24413=CARTESIAN_POINT('Ctrl Pts',(-2.1,-0.00329277923049777,6.87711561177094));
#24414=CARTESIAN_POINT('Ctrl Pts',(-2.1,0.00380833581134274,6.87777875025432));
#24415=CARTESIAN_POINT('Ctrl Pts',(-2.1,0.010934154274537,6.87828439261757));
#24416=CARTESIAN_POINT('Ctrl Pts',(-2.1,0.0180564268157742,6.87863124049195));
#24417=CARTESIAN_POINT('Ctrl Pts',(-2.1,0.0436614570733077,6.87987818102488));
#24418=CARTESIAN_POINT('Ctrl Pts',(-2.1,0.0692830486968658,6.87908401838085));
#24419=CARTESIAN_POINT('Ctrl Pts',(-2.1,0.0946701039420577,6.87627112264398));
#24420=CARTESIAN_POINT('Ctrl Pts',(-2.1,0.105116630998588,6.87511364332475));
#24421=CARTESIAN_POINT('Ctrl Pts',(-2.1,0.115523671677657,6.87361376587106));
#24422=CARTESIAN_POINT('Ctrl Pts',(-2.1,0.125874323021446,6.87177056809269));
#24423=CARTESIAN_POINT('Ctrl Pts',(-2.1,0.138413824297786,6.86953758969098));
#24424=CARTESIAN_POINT('Ctrl Pts',(-2.1,0.150870601134534,6.86680082502239));
#24425=CARTESIAN_POINT('Ctrl Pts',(-2.1,0.163219456840939,6.86357425405869));
#24426=CARTESIAN_POINT('Ctrl Pts',(-2.1,0.170695776276485,6.8616208038136));
#24427=CARTESIAN_POINT('Ctrl Pts',(-2.1,0.178132534318461,6.85948775559199));
#24428=CARTESIAN_POINT('Ctrl Pts',(-2.1,0.185524032856684,6.85717764382782));
#24429=CARTESIAN_POINT('Ctrl Pts',(-2.1,0.191333634449564,6.85536193231609));
#24430=CARTESIAN_POINT('Ctrl Pts',(-2.1,0.197115271577026,6.85343663586951));
#24431=CARTESIAN_POINT('Ctrl Pts',(-2.1,0.202852164838079,6.85140831852427));
#24432=CARTESIAN_POINT('Ctrl Pts',(-2.1,0.227408324506361,6.84272632248192));
#24433=CARTESIAN_POINT('Ctrl Pts',(-2.1,0.251209399850707,6.83214163505072));
#24434=CARTESIAN_POINT('Ctrl Pts',(-2.1,0.274050638756253,6.81980030995607));
#24435=CARTESIAN_POINT('Ctrl Pts',(-2.1,0.297081928279728,6.80735629881755));
#24436=CARTESIAN_POINT('Ctrl Pts',(-2.1,0.319138676313367,6.79312590368834));
#24437=CARTESIAN_POINT('Ctrl Pts',(-2.1,0.33999937244817,6.77720843590635));
#24438=CARTESIAN_POINT('Ctrl Pts',(-2.1,0.343569976374306,6.77448393560256));
#24439=CARTESIAN_POINT('Ctrl Pts',(-2.1,0.347105483833496,6.77170989850117));
#24440=CARTESIAN_POINT('Ctrl Pts',(-2.1,0.350604705166974,6.76888668926355));
#24441=CARTESIAN_POINT('Ctrl Pts',(-2.1,0.353884815611532,6.76624026103711));
#24442=CARTESIAN_POINT('Ctrl Pts',(-2.1,0.357133041678995,6.76355062538503));
#24443=CARTESIAN_POINT('Ctrl Pts',(-2.1,0.360348823959175,6.76081852140068));
#24444=CARTESIAN_POINT('Ctrl Pts',(-2.46703183294109,0.426306423912841,
6.39998913682467));
#24445=CARTESIAN_POINT('Ctrl Pts',(-2.46387625438919,0.426248106936643,
6.45633454115753));
#24446=CARTESIAN_POINT('Ctrl Pts',(-2.46072067583729,0.415012427400236,
6.51270250838063));
#24447=CARTESIAN_POINT('Ctrl Pts',(-2.45756509728538,0.39325469889476,6.56466465519153));
#24448=CARTESIAN_POINT('Ctrl Pts',(-2.45359215175999,0.365861221379708,
6.63008618574973));
#24449=CARTESIAN_POINT('Ctrl Pts',(-2.4496192062346,0.321788838359503,6.68852388050336));
#24450=CARTESIAN_POINT('Ctrl Pts',(-2.4456462607092,0.266417048735948,6.73284480312799));
#24451=CARTESIAN_POINT('Ctrl Pts',(-2.44167331518381,0.211045259112394,
6.77716572575262));
#24452=CARTESIAN_POINT('Ctrl Pts',(-2.43770036965842,0.144374062885491,
6.80736987624826));
#24453=CARTESIAN_POINT('Ctrl Pts',(-2.43372742413302,0.0745413820730864,
6.8197705196968));
#24454=CARTESIAN_POINT('Ctrl Pts',(-2.42975447860763,0.00470870126068151,
6.83217116314535));
#24455=CARTESIAN_POINT('Ctrl Pts',(-2.42578153308224,-0.0682854641372245,
6.82676829954679));
#24456=CARTESIAN_POINT('Ctrl Pts',(-2.42180858755684,-0.135531407000747,
6.80422140536676));
#24457=CARTESIAN_POINT('Ctrl Pts',(-2.41783564203145,-0.202777349864269,
6.78167451118673));
#24458=CARTESIAN_POINT('Ctrl Pts',(-2.41386269650606,-0.264275070193409,
6.74198358642523));
#24459=CARTESIAN_POINT('Ctrl Pts',(-2.40988975098066,-0.312518123176517,
6.68999332669579));
#24460=CARTESIAN_POINT('Ctrl Pts',(-2.40591680545527,-0.360761176159625,
6.63800306696635));
#24461=CARTESIAN_POINT('Ctrl Pts',(-2.40194385992988,-0.395749561796702,
6.57371347226898));
#24462=CARTESIAN_POINT('Ctrl Pts',(-2.39797091440449,-0.413212578910154,
6.50497176512118));
#24463=CARTESIAN_POINT('Ctrl Pts',(-2.39399796887909,-0.430675596023606,
6.43623005797338));
#24464=CARTESIAN_POINT('Ctrl Pts',(-2.3900250233537,-0.430613244613433,
6.36303623837515));
#24465=CARTESIAN_POINT('Ctrl Pts',(-2.38605207782831,-0.413033135329271,
6.29432438331576));
#24466=CARTESIAN_POINT('Ctrl Pts',(-2.38207913230291,-0.395453026045109,
6.22561252825636));
#24467=CARTESIAN_POINT('Ctrl Pts',(-2.37810618677752,-0.360355158886957,
6.16138263773582));
#24468=CARTESIAN_POINT('Ctrl Pts',(-2.37413324125213,-0.312023598397992,
6.10947464674327));
#24469=CARTESIAN_POINT('Ctrl Pts',(-2.37016029572673,-0.263692037909028,
6.05756665575072));
#24470=CARTESIAN_POINT('Ctrl Pts',(-2.36618735020134,-0.20212678408925,
6.01798056428618));
#24471=CARTESIAN_POINT('Ctrl Pts',(-2.36221440467595,-0.1348425249389,5.99554827196608));
#24472=CARTESIAN_POINT('Ctrl Pts',(-2.35824145915055,-0.0675582657885491,
5.97311597964598));
#24473=CARTESIAN_POINT('Ctrl Pts',(-2.35426851362516,0.00544499869237483,
5.96783748647033));
#24474=CARTESIAN_POINT('Ctrl Pts',(-2.35029556809977,0.0752564507749232,
5.98035708815828));
#24475=CARTESIAN_POINT('Ctrl Pts',(-2.34632262257437,0.145067902857471,
5.99287668984623));
#24476=CARTESIAN_POINT('Ctrl Pts',(-2.34234967704898,0.211687542541645,
6.02319438639778));
#24477=CARTESIAN_POINT('Ctrl Pts',(-2.33837673152359,0.266983740765077,
6.06760958345802));
#24478=CARTESIAN_POINT('Ctrl Pts',(-2.33440378599819,0.322279938988509,
6.11202478051826));
#24479=CARTESIAN_POINT('Ctrl Pts',(-2.3304308404728,0.366252695751201,6.17053747808719));
#24480=CARTESIAN_POINT('Ctrl Pts',(-2.32645789494741,0.393534672723127,
6.236005584836));
#24481=CARTESIAN_POINT('Ctrl Pts',(-2.32331587427864,0.415110738889366,
6.28778131224916));
#24482=CARTESIAN_POINT('Ctrl Pts',(-2.32017385360987,0.4262475506417,6.34390730291496));
#24483=CARTESIAN_POINT('Ctrl Pts',(-2.31703183294109,0.426305653513777,
6.40001091236462));
#24484=CARTESIAN_POINT('Ctrl Pts',(-2.6,0.132288496556895,5.90755938055567));
#24485=CARTESIAN_POINT('Ctrl Pts',(-2.6,0.157089924837099,5.91642640455182));
#24486=CARTESIAN_POINT('Ctrl Pts',(-2.6,0.181088073064976,5.9272189255245));
#24487=CARTESIAN_POINT('Ctrl Pts',(-2.6,0.204091900162786,5.93978802247808));
#24488=CARTESIAN_POINT('Ctrl Pts',(-2.6,0.226981614101412,5.95229476896469));
#24489=CARTESIAN_POINT('Ctrl Pts',(-2.6,0.248887897831876,5.96656143458844));
#24490=CARTESIAN_POINT('Ctrl Pts',(-2.6,0.269590200964406,5.98248076289354));
#24491=CARTESIAN_POINT('Ctrl Pts',(-2.6,0.276528918772376,5.98781638792494));
#24492=CARTESIAN_POINT('Ctrl Pts',(-2.6,0.283332046569503,5.99333793609881));
#24493=CARTESIAN_POINT('Ctrl Pts',(-2.6,0.289990147837974,5.99904209573216));
#24494=CARTESIAN_POINT('Ctrl Pts',(-2.6,0.296028106433828,6.00421496383698));
#24495=CARTESIAN_POINT('Ctrl Pts',(-2.6,0.301949771037903,6.00954116989861));
#24496=CARTESIAN_POINT('Ctrl Pts',(-2.6,0.307727671725424,6.01499858003089));
#24497=CARTESIAN_POINT('Ctrl Pts',(-2.6,0.318182122624537,6.02487313990129));
#24498=CARTESIAN_POINT('Ctrl Pts',(-2.6,0.32817930410564,6.03518740593773));
#24499=CARTESIAN_POINT('Ctrl Pts',(-2.6,0.337684947200095,6.04592058651842));
#24500=CARTESIAN_POINT('Ctrl Pts',(-2.6,0.35463663907465,6.06506138196275));
#24501=CARTESIAN_POINT('Ctrl Pts',(-2.6,0.370027957593029,6.08553349763026));
#24502=CARTESIAN_POINT('Ctrl Pts',(-2.6,0.383735216002276,6.10712564152075));
#24503=CARTESIAN_POINT('Ctrl Pts',(-2.6,0.39189872132373,6.11998507528124));
#24504=CARTESIAN_POINT('Ctrl Pts',(-2.6,0.399464029634324,6.13324224816933));
#24505=CARTESIAN_POINT('Ctrl Pts',(-2.6,0.406396423774992,6.1468545793287));
#24506=CARTESIAN_POINT('Ctrl Pts',(-2.6,0.409857954474058,6.15365158210118));
#24507=CARTESIAN_POINT('Ctrl Pts',(-2.6,0.413162930739684,6.16054073803517));
#24508=CARTESIAN_POINT('Ctrl Pts',(-2.6,0.416296070484027,6.16749212337976));
#24509=CARTESIAN_POINT('Ctrl Pts',(-2.6,0.426533299061843,6.19020509710957));
#24510=CARTESIAN_POINT('Ctrl Pts',(-2.6,0.434966161858725,6.21362881910558));
#24511=CARTESIAN_POINT('Ctrl Pts',(-2.6,0.441477406647537,6.23756556523482));
#24512=CARTESIAN_POINT('Ctrl Pts',(-2.6,0.443239379224161,6.24404295805621));
#24513=CARTESIAN_POINT('Ctrl Pts',(-2.6,0.444860350146518,6.25055797543335));
#24514=CARTESIAN_POINT('Ctrl Pts',(-2.6,0.44633733619218,6.25710677385474));
#24515=CARTESIAN_POINT('Ctrl Pts',(-2.6,0.450544524902758,6.27576099937518));
#24516=CARTESIAN_POINT('Ctrl Pts',(-2.6,0.453584703119787,6.29468965910361));
#24517=CARTESIAN_POINT('Ctrl Pts',(-2.6,0.455444326288054,6.31378084410223));
#24518=CARTESIAN_POINT('Ctrl Pts',(-2.6,0.456025440853221,6.31974665796081));
#24519=CARTESIAN_POINT('Ctrl Pts',(-2.6,0.456491144811005,6.32572830613997));
#24520=CARTESIAN_POINT('Ctrl Pts',(-2.6,0.456840676091559,6.33172224529114));
#24521=CARTESIAN_POINT('Ctrl Pts',(-2.6,0.457162778165346,6.33724581453417));
#24522=CARTESIAN_POINT('Ctrl Pts',(-2.6,0.457385661676131,6.34277019876787));
#24523=CARTESIAN_POINT('Ctrl Pts',(-2.6,0.457509644065614,6.34829248285953));
#24524=CARTESIAN_POINT('Ctrl Pts',(-2.6,0.458052816417877,6.37248585461552));
#24525=CARTESIAN_POINT('Ctrl Pts',(-2.6,0.456701759624391,6.39664121290135));
#24526=CARTESIAN_POINT('Ctrl Pts',(-2.6,0.453453339531317,6.42053138158929));
#24527=CARTESIAN_POINT('Ctrl Pts',(-2.6,0.450523324248874,6.44207987511851));
#24528=CARTESIAN_POINT('Ctrl Pts',(-2.6,0.446048919178311,6.46341331208366));
#24529=CARTESIAN_POINT('Ctrl Pts',(-2.6,0.439994176553064,6.48435098741415));
#24530=CARTESIAN_POINT('Ctrl Pts',(-2.6,0.438094472520504,6.49092028172105));
#24531=CARTESIAN_POINT('Ctrl Pts',(-2.6,0.436038962655861,6.4974504658391));
#24532=CARTESIAN_POINT('Ctrl Pts',(-2.6,0.43382941905493,6.50393615250028));
#24533=CARTESIAN_POINT('Ctrl Pts',(-2.6,0.431714290768034,6.5101447013206));
#24534=CARTESIAN_POINT('Ctrl Pts',(-2.6,0.42946061872238,6.5163046335942));
#24535=CARTESIAN_POINT('Ctrl Pts',(-2.6,0.427072414698455,6.5224077707279));
#24536=CARTESIAN_POINT('Ctrl Pts',(-2.6,0.421492488317325,6.53666746360122));
#24537=CARTESIAN_POINT('Ctrl Pts',(-2.6,0.415176231857449,6.5506245268354));
#24538=CARTESIAN_POINT('Ctrl Pts',(-2.6,0.408152204549093,6.56422236660796));
#24539=CARTESIAN_POINT('Ctrl Pts',(-2.6,0.402591346359437,6.57498765201209));
#24540=CARTESIAN_POINT('Ctrl Pts',(-2.6,0.396586710322636,6.58552771963742));
#24541=CARTESIAN_POINT('Ctrl Pts',(-2.6,0.390149689096489,6.59581166017504));
#24542=CARTESIAN_POINT('Ctrl Pts',(-2.6,0.386403333843806,6.6017969277853));
#24543=CARTESIAN_POINT('Ctrl Pts',(-2.6,0.382511806820547,6.60769294534655));
#24544=CARTESIAN_POINT('Ctrl Pts',(-2.6,0.378483683496843,6.61348517016826));
#24545=CARTESIAN_POINT('Ctrl Pts',(-2.6,0.365269544048599,6.63248639241469));
#24546=CARTESIAN_POINT('Ctrl Pts',(-2.6,0.350570496167934,6.65040177272496));
#24547=CARTESIAN_POINT('Ctrl Pts',(-2.6,0.334470605331163,6.66701291851188));
#24548=CARTESIAN_POINT('Ctrl Pts',(-2.6,0.332980284132811,6.66855056512987));
#24549=CARTESIAN_POINT('Ctrl Pts',(-2.6,0.331477939680677,6.67007700481367));
#24550=CARTESIAN_POINT('Ctrl Pts',(-2.6,0.329963627179693,6.67159204424712));
#24551=CARTESIAN_POINT('Ctrl Pts',(-2.6,0.327462974104075,6.67409389773937));
#24552=CARTESIAN_POINT('Ctrl Pts',(-2.6,0.324929685151723,6.67656466471947));
#24553=CARTESIAN_POINT('Ctrl Pts',(-2.6,0.322364416527274,6.67900379523474));
#24554=CARTESIAN_POINT('Origin',(2.35,0.,6.4));
#24555=CARTESIAN_POINT('Origin',(2.1,0.,6.4));
#24556=CARTESIAN_POINT('',(2.1,-0.4,6.4));
#24557=CARTESIAN_POINT('Origin',(2.1,0.,6.4));
#24558=CARTESIAN_POINT('Origin',(1.9,0.,6.4));
#24559=CARTESIAN_POINT('',(1.2,-0.4,6.4));
#24560=CARTESIAN_POINT('',(1.9,-0.4,6.4));
#24561=CARTESIAN_POINT('Origin',(1.2,0.,6.4));
#24562=CARTESIAN_POINT('Origin',(1.2,0.,6.4));
#24563=CARTESIAN_POINT('',(1.2,-0.2,6.4));
#24564=CARTESIAN_POINT('Origin',(1.2,0.,6.4));
#24565=CARTESIAN_POINT('Origin',(1.55,0.,6.4));
#24566=CARTESIAN_POINT('',(0.565685424949238,-0.2,6.4));
#24567=CARTESIAN_POINT('',(1.55,-0.2,6.4));
#24568=CARTESIAN_POINT('',(0.565685424949238,0.2,6.4));
#24569=CARTESIAN_POINT('Ctrl Pts',(0.565685424949238,0.2,6.4));
#24570=CARTESIAN_POINT('Ctrl Pts',(0.565685424949238,0.2,6.42532921208158));
#24571=CARTESIAN_POINT('Ctrl Pts',(0.567565356574251,0.194898067853762,
6.45220039469271));
#24572=CARTESIAN_POINT('Ctrl Pts',(0.574186082552466,0.17443058152527,6.50141063599154));
#24573=CARTESIAN_POINT('Ctrl Pts',(0.578813771212597,0.159074095999941,
6.52376861647468));
#24574=CARTESIAN_POINT('Ctrl Pts',(0.587374622031365,0.123776803829002,
6.55906590864562));
#24575=CARTESIAN_POINT('Ctrl Pts',(0.59188739106068,0.101415562391481,6.57442869722332));
#24576=CARTESIAN_POINT('Ctrl Pts',(0.598240475886912,0.0521932274441716,
6.59490088416061));
#24577=CARTESIAN_POINT('Ctrl Pts',(0.6,0.0253174643734703,6.6));
#24578=CARTESIAN_POINT('Ctrl Pts',(0.6,-0.0253174643734703,6.6));
#24579=CARTESIAN_POINT('Ctrl Pts',(0.598240475886912,-0.0521932274441708,
6.59490088416061));
#24580=CARTESIAN_POINT('Ctrl Pts',(0.59188739106068,-0.10141556239148,6.57442869722332));
#24581=CARTESIAN_POINT('Ctrl Pts',(0.587374622031365,-0.123776803829002,
6.55906590864562));
#24582=CARTESIAN_POINT('Ctrl Pts',(0.578813771212597,-0.159074095999941,
6.52376861647468));
#24583=CARTESIAN_POINT('Ctrl Pts',(0.574186082552466,-0.17443058152527,
6.50141063599154));
#24584=CARTESIAN_POINT('Ctrl Pts',(0.567565356574251,-0.194898067853762,
6.45220039469271));
#24585=CARTESIAN_POINT('Ctrl Pts',(0.565685424949238,-0.2,6.42532921208158));
#24586=CARTESIAN_POINT('Ctrl Pts',(0.565685424949238,-0.2,6.4));
#24587=CARTESIAN_POINT('Ctrl Pts',(0.565685424949238,-0.2,6.4));
#24588=CARTESIAN_POINT('Ctrl Pts',(0.565685424949238,-0.2,6.37467078791842));
#24589=CARTESIAN_POINT('Ctrl Pts',(0.567565356574251,-0.194898067853762,
6.3477996053073));
#24590=CARTESIAN_POINT('Ctrl Pts',(0.574186082552466,-0.17443058152527,
6.29858936400846));
#24591=CARTESIAN_POINT('Ctrl Pts',(0.578813771212597,-0.159074095999941,
6.27623138352532));
#24592=CARTESIAN_POINT('Ctrl Pts',(0.587374622031365,-0.123776803829002,
6.24093409135438));
#24593=CARTESIAN_POINT('Ctrl Pts',(0.59188739106068,-0.101415562391481,
6.22557130277668));
#24594=CARTESIAN_POINT('Ctrl Pts',(0.598240475886912,-0.0521932274441716,
6.20509911583939));
#24595=CARTESIAN_POINT('Ctrl Pts',(0.6,-0.0253174643734704,6.2));
#24596=CARTESIAN_POINT('Ctrl Pts',(0.6,0.0253174643734703,6.2));
#24597=CARTESIAN_POINT('Ctrl Pts',(0.598240475886912,0.0521932274441716,
6.20509911583939));
#24598=CARTESIAN_POINT('Ctrl Pts',(0.59188739106068,0.101415562391481,6.22557130277668));
#24599=CARTESIAN_POINT('Ctrl Pts',(0.587374622031365,0.123776803829002,
6.24093409135438));
#24600=CARTESIAN_POINT('Ctrl Pts',(0.578813771212597,0.159074095999941,
6.27623138352532));
#24601=CARTESIAN_POINT('Ctrl Pts',(0.574186082552466,0.17443058152527,6.29858936400846));
#24602=CARTESIAN_POINT('Ctrl Pts',(0.567565356574251,0.194898067853762,
6.3477996053073));
#24603=CARTESIAN_POINT('Ctrl Pts',(0.565685424949238,0.2,6.37467078791842));
#24604=CARTESIAN_POINT('Ctrl Pts',(0.565685424949238,0.2,6.4));
#24605=CARTESIAN_POINT('Origin',(2.,0.,6.4));
#24606=CARTESIAN_POINT('',(2.37276210354093,0.3605551275464,5.8));
#24607=CARTESIAN_POINT('',(2.6,0.3605551275464,5.8));
#24608=CARTESIAN_POINT('',(2.,0.3605551275464,5.8));
#24609=CARTESIAN_POINT('Ctrl Pts',(2.33023603954621,0.574456264653803,6.8));
#24610=CARTESIAN_POINT('Ctrl Pts',(2.3232708588146,0.602709964998632,6.75942371209316));
#24611=CARTESIAN_POINT('Ctrl Pts',(2.31670997613269,0.627102242782997,6.71508313975596));
#24612=CARTESIAN_POINT('Ctrl Pts',(2.30129622342295,0.682214955011516,6.58244341832651));
#24613=CARTESIAN_POINT('Ctrl Pts',(2.2956480566498,0.7,6.48846273735544));
#24614=CARTESIAN_POINT('Ctrl Pts',(2.2956480566498,0.7,6.4));
#24615=CARTESIAN_POINT('Ctrl Pts',(2.2956480566498,0.7,6.31153726264456));
#24616=CARTESIAN_POINT('Ctrl Pts',(2.30129622342295,0.682214955011516,6.21755658167349));
#24617=CARTESIAN_POINT('Ctrl Pts',(2.32131846716735,0.610624332115547,6.04525948552425));
#24618=CARTESIAN_POINT('Ctrl Pts',(2.3353634864858,0.556843997628587,5.96689450396742));
#24619=CARTESIAN_POINT('Ctrl Pts',(2.35662323311261,0.455977300410207,5.86602780674904));
#24620=CARTESIAN_POINT('Ctrl Pts',(2.36516699585665,0.410537452879607,5.83003563947597));
#24621=CARTESIAN_POINT('Ctrl Pts',(2.37276210354093,0.3605551275464,5.8));
#24622=CARTESIAN_POINT('Origin',(2.,0.,6.4));
#24623=CARTESIAN_POINT('',(2.37276210354093,-0.3605551275464,5.8));
#24624=CARTESIAN_POINT('Ctrl Pts',(2.37276210354093,-0.3605551275464,5.8));
#24625=CARTESIAN_POINT('Ctrl Pts',(2.36516699585665,-0.410537452879608,
5.83003563947597));
#24626=CARTESIAN_POINT('Ctrl Pts',(2.35662323311261,-0.455977300410207,
5.86602780674904));
#24627=CARTESIAN_POINT('Ctrl Pts',(2.3353634864858,-0.556843997628587,5.96689450396742));
#24628=CARTESIAN_POINT('Ctrl Pts',(2.32131846716735,-0.610624332115547,
6.04525948552425));
#24629=CARTESIAN_POINT('Ctrl Pts',(2.30129622342295,-0.682214955011516,
6.21755658167349));
#24630=CARTESIAN_POINT('Ctrl Pts',(2.2956480566498,-0.7,6.31153726264456));
#24631=CARTESIAN_POINT('Ctrl Pts',(2.2956480566498,-0.7,6.48846273735544));
#24632=CARTESIAN_POINT('Ctrl Pts',(2.30129622342295,-0.682214955011516,
6.58244341832651));
#24633=CARTESIAN_POINT('Ctrl Pts',(2.31670997613269,-0.627102242782997,
6.71508313975596));
#24634=CARTESIAN_POINT('Ctrl Pts',(2.3232708588146,-0.602709964998632,6.75942371209315));
#24635=CARTESIAN_POINT('Ctrl Pts',(2.33023603954621,-0.574456264653803,
6.8));
#24636=CARTESIAN_POINT('',(2.6,-0.3605551275464,5.8));
#24637=CARTESIAN_POINT('',(2.,-0.3605551275464,5.8));
#24638=CARTESIAN_POINT('Origin',(2.6,0.,6.4));
#24639=CARTESIAN_POINT('Origin',(2.,0.,6.4));
#24640=CARTESIAN_POINT('Origin',(2.6,0.,6.4));
#24641=CARTESIAN_POINT('',(2.6,0.,5.8));
#24642=CARTESIAN_POINT('Origin',(0.,0.,5.8));
#24643=CARTESIAN_POINT('',(-4.,2.8,5.8));
#24644=CARTESIAN_POINT('',(-4.,-2.8,5.8));
#24645=CARTESIAN_POINT('',(-4.,2.8,5.8));
#24646=CARTESIAN_POINT('',(4.,-2.8,5.8));
#24647=CARTESIAN_POINT('',(-4.,-2.8,5.8));
#24648=CARTESIAN_POINT('',(4.,2.8,5.8));
#24649=CARTESIAN_POINT('',(4.,-2.8,5.8));
#24650=CARTESIAN_POINT('',(4.,2.8,5.8));
#24651=CARTESIAN_POINT('',(3.35,-2.4,5.8));
#24652=CARTESIAN_POINT('Origin',(3.6,-2.4,5.8));
#24653=CARTESIAN_POINT('',(-3.85,-2.4,5.8));
#24654=CARTESIAN_POINT('Origin',(-3.6,-2.4,5.8));
#24655=CARTESIAN_POINT('',(-3.85,2.4,5.8));
#24656=CARTESIAN_POINT('Origin',(-3.6,2.4,5.8));
#24657=CARTESIAN_POINT('',(3.35,2.4,5.8));
#24658=CARTESIAN_POINT('Origin',(3.6,2.4,5.8));
#24659=CARTESIAN_POINT('',(-2.37276210354093,-0.3605551275464,5.8));
#24660=CARTESIAN_POINT('Origin',(0.,0.,5.8));
#24661=CARTESIAN_POINT('',(-2.6,-0.3605551275464,5.8));
#24662=CARTESIAN_POINT('',(-2.,-0.3605551275464,5.8));
#24663=CARTESIAN_POINT('',(-2.6,0.3605551275464,5.8));
#24664=CARTESIAN_POINT('',(-2.6,0.,5.8));
#24665=CARTESIAN_POINT('',(-2.37276210354093,0.3605551275464,5.8));
#24666=CARTESIAN_POINT('',(-2.,0.3605551275464,5.8));
#24667=CARTESIAN_POINT('Origin',(0.,0.,5.8));
#24668=CARTESIAN_POINT('Origin',(0.,0.,5.8));
#24669=CARTESIAN_POINT('Ctrl Pts',(-2.33023603954621,-0.574456264653803,
6.8));
#24670=CARTESIAN_POINT('Ctrl Pts',(-2.3232708588146,-0.602709964998632,
6.75942371209316));
#24671=CARTESIAN_POINT('Ctrl Pts',(-2.31670997613269,-0.627102242782997,
6.71508313975596));
#24672=CARTESIAN_POINT('Ctrl Pts',(-2.30129622342295,-0.682214955011516,
6.58244341832651));
#24673=CARTESIAN_POINT('Ctrl Pts',(-2.2956480566498,-0.7,6.48846273735544));
#24674=CARTESIAN_POINT('Ctrl Pts',(-2.2956480566498,-0.7,6.4));
#24675=CARTESIAN_POINT('Ctrl Pts',(-2.2956480566498,-0.7,6.31153726264456));
#24676=CARTESIAN_POINT('Ctrl Pts',(-2.30129622342295,-0.682214955011516,
6.21755658167349));
#24677=CARTESIAN_POINT('Ctrl Pts',(-2.32131846716735,-0.610624332115547,
6.04525948552425));
#24678=CARTESIAN_POINT('Ctrl Pts',(-2.3353634864858,-0.556843997628587,
5.96689450396742));
#24679=CARTESIAN_POINT('Ctrl Pts',(-2.35662323311261,-0.455977300410207,
5.86602780674904));
#24680=CARTESIAN_POINT('Ctrl Pts',(-2.36516699585665,-0.410537452879607,
5.83003563947597));
#24681=CARTESIAN_POINT('Ctrl Pts',(-2.37276210354093,-0.3605551275464,5.8));
#24682=CARTESIAN_POINT('Origin',(-2.35,0.,6.4));
#24683=CARTESIAN_POINT('Origin',(-2.1,0.,6.4));
#24684=CARTESIAN_POINT('',(-2.1,0.4,6.4));
#24685=CARTESIAN_POINT('Origin',(-2.1,0.,6.4));
#24686=CARTESIAN_POINT('Origin',(-1.9,0.,6.4));
#24687=CARTESIAN_POINT('',(-1.2,0.4,6.4));
#24688=CARTESIAN_POINT('',(-1.9,0.4,6.4));
#24689=CARTESIAN_POINT('Origin',(-1.2,0.,6.4));
#24690=CARTESIAN_POINT('Origin',(-1.2,0.,6.4));
#24691=CARTESIAN_POINT('',(-1.2,0.2,6.4));
#24692=CARTESIAN_POINT('Origin',(-1.2,0.,6.4));
#24693=CARTESIAN_POINT('Origin',(-1.55,0.,6.4));
#24694=CARTESIAN_POINT('',(-0.565685424949238,0.2,6.4));
#24695=CARTESIAN_POINT('',(-1.55,0.2,6.4));
#24696=CARTESIAN_POINT('',(-0.6,1.93921692146525E-17,6.6));
#24697=CARTESIAN_POINT('Ctrl Pts',(-0.6,-2.77555756156289E-17,6.6));
#24698=CARTESIAN_POINT('Ctrl Pts',(-0.6,0.0253174643734703,6.6));
#24699=CARTESIAN_POINT('Ctrl Pts',(-0.598240475886912,0.0521932274441708,
6.59490088416061));
#24700=CARTESIAN_POINT('Ctrl Pts',(-0.59188739106068,0.10141556239148,6.57442869722332));
#24701=CARTESIAN_POINT('Ctrl Pts',(-0.587374622031365,0.123776803829002,
6.55906590864562));
#24702=CARTESIAN_POINT('Ctrl Pts',(-0.578813771212597,0.159074095999941,
6.52376861647468));
#24703=CARTESIAN_POINT('Ctrl Pts',(-0.574186082552466,0.17443058152527,
6.50141063599154));
#24704=CARTESIAN_POINT('Ctrl Pts',(-0.567565356574251,0.194898067853762,
6.45220039469271));
#24705=CARTESIAN_POINT('Ctrl Pts',(-0.565685424949238,0.2,6.42532921208158));
#24706=CARTESIAN_POINT('Ctrl Pts',(-0.565685424949238,0.2,6.4));
#24707=CARTESIAN_POINT('',(-0.565685424949238,-0.2,6.4));
#24708=CARTESIAN_POINT('Ctrl Pts',(-0.565685424949238,-0.2,6.4));
#24709=CARTESIAN_POINT('Ctrl Pts',(-0.565685424949238,-0.2,6.42532921208158));
#24710=CARTESIAN_POINT('Ctrl Pts',(-0.567565356574251,-0.194898067853762,
6.45220039469271));
#24711=CARTESIAN_POINT('Ctrl Pts',(-0.574186082552466,-0.17443058152527,
6.50141063599154));
#24712=CARTESIAN_POINT('Ctrl Pts',(-0.578813771212597,-0.159074095999941,
6.52376861647468));
#24713=CARTESIAN_POINT('Ctrl Pts',(-0.587374622031365,-0.123776803829002,
6.55906590864562));
#24714=CARTESIAN_POINT('Ctrl Pts',(-0.59188739106068,-0.101415562391481,
6.57442869722332));
#24715=CARTESIAN_POINT('Ctrl Pts',(-0.598240475886912,-0.0521932274441716,
6.59490088416061));
#24716=CARTESIAN_POINT('Ctrl Pts',(-0.6,-0.0253174643734703,6.6));
#24717=CARTESIAN_POINT('Ctrl Pts',(-0.6,2.08166817117217E-17,6.6));
#24718=CARTESIAN_POINT('',(-0.6,1.59227222626989E-17,6.2));
#24719=CARTESIAN_POINT('Ctrl Pts',(-0.6,-4.85722573273506E-17,6.2));
#24720=CARTESIAN_POINT('Ctrl Pts',(-0.6,-0.0253174643734703,6.2));
#24721=CARTESIAN_POINT('Ctrl Pts',(-0.598240475886912,-0.0521932274441716,
6.20509911583939));
#24722=CARTESIAN_POINT('Ctrl Pts',(-0.59188739106068,-0.101415562391481,
6.22557130277668));
#24723=CARTESIAN_POINT('Ctrl Pts',(-0.587374622031365,-0.123776803829002,
6.24093409135438));
#24724=CARTESIAN_POINT('Ctrl Pts',(-0.578813771212597,-0.159074095999941,
6.27623138352532));
#24725=CARTESIAN_POINT('Ctrl Pts',(-0.574186082552466,-0.17443058152527,
6.29858936400846));
#24726=CARTESIAN_POINT('Ctrl Pts',(-0.567565356574251,-0.194898067853762,
6.3477996053073));
#24727=CARTESIAN_POINT('Ctrl Pts',(-0.565685424949238,-0.2,6.37467078791842));
#24728=CARTESIAN_POINT('Ctrl Pts',(-0.565685424949238,-0.2,6.4));
#24729=CARTESIAN_POINT('Ctrl Pts',(-0.565685424949238,0.2,6.4));
#24730=CARTESIAN_POINT('Ctrl Pts',(-0.565685424949238,0.2,6.37467078791842));
#24731=CARTESIAN_POINT('Ctrl Pts',(-0.567565356574251,0.194898067853762,
6.3477996053073));
#24732=CARTESIAN_POINT('Ctrl Pts',(-0.574186082552466,0.17443058152527,
6.29858936400846));
#24733=CARTESIAN_POINT('Ctrl Pts',(-0.578813771212597,0.159074095999941,
6.27623138352532));
#24734=CARTESIAN_POINT('Ctrl Pts',(-0.587374622031365,0.123776803829002,
6.24093409135438));
#24735=CARTESIAN_POINT('Ctrl Pts',(-0.59188739106068,0.101415562391481,
6.22557130277668));
#24736=CARTESIAN_POINT('Ctrl Pts',(-0.598240475886912,0.0521932274441716,
6.20509911583939));
#24737=CARTESIAN_POINT('Ctrl Pts',(-0.6,0.0253174643734703,6.2));
#24738=CARTESIAN_POINT('Ctrl Pts',(-0.6,-2.77555756156289E-17,6.2));
#24739=CARTESIAN_POINT('Origin',(-2.6,0.,6.4));
#24740=CARTESIAN_POINT('Origin',(-2.6,0.,6.4));
#24741=CARTESIAN_POINT('Origin',(-2.,0.,6.4));
#24742=CARTESIAN_POINT('Ctrl Pts',(-2.37276210354093,0.3605551275464,5.8));
#24743=CARTESIAN_POINT('Ctrl Pts',(-2.36516699585665,0.410537452879608,
5.83003563947597));
#24744=CARTESIAN_POINT('Ctrl Pts',(-2.35662323311261,0.455977300410207,
5.86602780674904));
#24745=CARTESIAN_POINT('Ctrl Pts',(-2.3353634864858,0.556843997628587,5.96689450396742));
#24746=CARTESIAN_POINT('Ctrl Pts',(-2.32131846716735,0.610624332115547,
6.04525948552425));
#24747=CARTESIAN_POINT('Ctrl Pts',(-2.30129622342295,0.682214955011516,
6.21755658167349));
#24748=CARTESIAN_POINT('Ctrl Pts',(-2.2956480566498,0.7,6.31153726264456));
#24749=CARTESIAN_POINT('Ctrl Pts',(-2.2956480566498,0.7,6.48846273735544));
#24750=CARTESIAN_POINT('Ctrl Pts',(-2.30129622342295,0.682214955011516,
6.58244341832651));
#24751=CARTESIAN_POINT('Ctrl Pts',(-2.31670997613269,0.627102242782997,
6.71508313975596));
#24752=CARTESIAN_POINT('Ctrl Pts',(-2.3232708588146,0.602709964998632,6.75942371209315));
#24753=CARTESIAN_POINT('Ctrl Pts',(-2.33023603954621,0.574456264653803,
6.8));
#24754=CARTESIAN_POINT('Origin',(0.,0.,5.8));
#24755=CARTESIAN_POINT('Origin',(3.6,-2.4,5.5));
#24756=CARTESIAN_POINT('',(3.35,-2.4,5.2));
#24757=CARTESIAN_POINT('',(3.35,-2.4,5.5));
#24758=CARTESIAN_POINT('Origin',(3.6,-2.4,5.2));
#24759=CARTESIAN_POINT('Origin',(-3.6,-2.4,5.5));
#24760=CARTESIAN_POINT('',(-3.85,-2.4,5.2));
#24761=CARTESIAN_POINT('',(-3.85,-2.4,5.5));
#24762=CARTESIAN_POINT('Origin',(-3.6,-2.4,5.2));
#24763=CARTESIAN_POINT('Origin',(-3.6,2.4,5.5));
#24764=CARTESIAN_POINT('',(-3.85,2.4,5.2));
#24765=CARTESIAN_POINT('',(-3.85,2.4,5.5));
#24766=CARTESIAN_POINT('Origin',(-3.6,2.4,5.2));
#24767=CARTESIAN_POINT('Origin',(3.6,2.4,5.5));
#24768=CARTESIAN_POINT('',(3.35,2.4,5.2));
#24769=CARTESIAN_POINT('',(3.35,2.4,5.5));
#24770=CARTESIAN_POINT('Origin',(3.6,2.4,5.2));
#24771=CARTESIAN_POINT('Origin',(0.,0.,5.5));
#24772=CARTESIAN_POINT('',(-0.6,7.34788079488412E-17,5.5));
#24773=CARTESIAN_POINT('',(-0.6,7.34788079488412E-17,5.2));
#24774=CARTESIAN_POINT('',(-0.6,7.34788079488412E-17,5.5));
#24775=CARTESIAN_POINT('Origin',(0.,0.,5.2));
#24776=CARTESIAN_POINT('Origin',(4.,2.8,5.2));
#24777=CARTESIAN_POINT('',(4.,2.8,5.2));
#24778=CARTESIAN_POINT('',(-4.,2.8,5.2));
#24779=CARTESIAN_POINT('',(4.,2.8,5.2));
#24780=CARTESIAN_POINT('',(-4.,2.8,5.2));
#24781=CARTESIAN_POINT('',(4.,2.8,5.2));
#24782=CARTESIAN_POINT('Origin',(4.,-2.8,5.2));
#24783=CARTESIAN_POINT('',(4.,-2.8,5.2));
#24784=CARTESIAN_POINT('',(4.,-2.8,5.2));
#24785=CARTESIAN_POINT('',(4.,-2.8,5.2));
#24786=CARTESIAN_POINT('Origin',(-4.,-2.8,5.2));
#24787=CARTESIAN_POINT('',(-4.,-2.8,5.2));
#24788=CARTESIAN_POINT('',(-4.,-2.8,5.2));
#24789=CARTESIAN_POINT('',(-4.,-2.8,5.2));
#24790=CARTESIAN_POINT('Origin',(-4.,2.8,5.2));
#24791=CARTESIAN_POINT('',(-4.,2.8,5.2));
#24792=CARTESIAN_POINT('Origin',(0.,0.,5.2));
#43945=UNCERTAINTY_MEASURE_WITH_UNIT(LENGTH_MEASURE(0.001),#43981,
'DISTANCE_ACCURACY_VALUE',
'Maximum model space distance between geometric entities at asserted c
onnectivities');
#43961=UNCERTAINTY_MEASURE_WITH_UNIT(LENGTH_MEASURE(0.001),#43981,
'DISTANCE_ACCURACY_VALUE',
'Maximum model space distance between geometric entities at asserted c
onnectivities');
#43964=(
GEOMETRIC_REPRESENTATION_CONTEXT(3)
GLOBAL_UNCERTAINTY_ASSIGNED_CONTEXT((#43945))
GLOBAL_UNIT_ASSIGNED_CONTEXT((#43981,#43983,#43984))
REPRESENTATION_CONTEXT('','3D')
);
#43980=(
GEOMETRIC_REPRESENTATION_CONTEXT(3)
GLOBAL_UNCERTAINTY_ASSIGNED_CONTEXT((#43961))
GLOBAL_UNIT_ASSIGNED_CONTEXT((#43981,#43983,#43984))
REPRESENTATION_CONTEXT('','3D')
);
#43981=(
LENGTH_UNIT()
NAMED_UNIT(*)
SI_UNIT(.CENTI.,.METRE.)
);
#43983=(
NAMED_UNIT(*)
PLANE_ANGLE_UNIT()
SI_UNIT($,.RADIAN.)
);
#43984=(
NAMED_UNIT(*)
SI_UNIT($,.STERADIAN.)
SOLID_ANGLE_UNIT()
);
#43987=SHAPE_DEFINITION_REPRESENTATION(#44005,#44057);
#44005=PRODUCT_DEFINITION_SHAPE('',$,#44076);
#44057=SHAPE_REPRESENTATION('',(#11636),#43964);
#44073=PRODUCT_DEFINITION_CONTEXT('part definition',#44129,'design');
#44076=PRODUCT_DEFINITION('Housing cover','Housing cover',#44094,#44073);
#44094=PRODUCT_DEFINITION_FORMATION('',$,#44133);
#44129=APPLICATION_CONTEXT(
'Core Data for Automotive Mechanical Design Process');
#44130=PRODUCT_CONTEXT('part definition',#44129,'mechanical');
#44133=PRODUCT('Housing cover','Housing cover',$,(#44130));
#44151=PRESENTATION_STYLE_ASSIGNMENT((#44163));
#44163=SURFACE_STYLE_USAGE(.BOTH.,#44175);
#44175=SURFACE_SIDE_STYLE('',(#44187));
#44187=SURFACE_STYLE_FILL_AREA(#44199);
#44199=FILL_AREA_STYLE('Sky blue',(#44211));
#44211=FILL_AREA_STYLE_COLOUR('Sky blue',#44223);
#44223=COLOUR_RGB('Sky blue',0.317647058823529,0.686274509803922,0.890196078431372);
ENDSEC;
END-ISO-10303-21;
